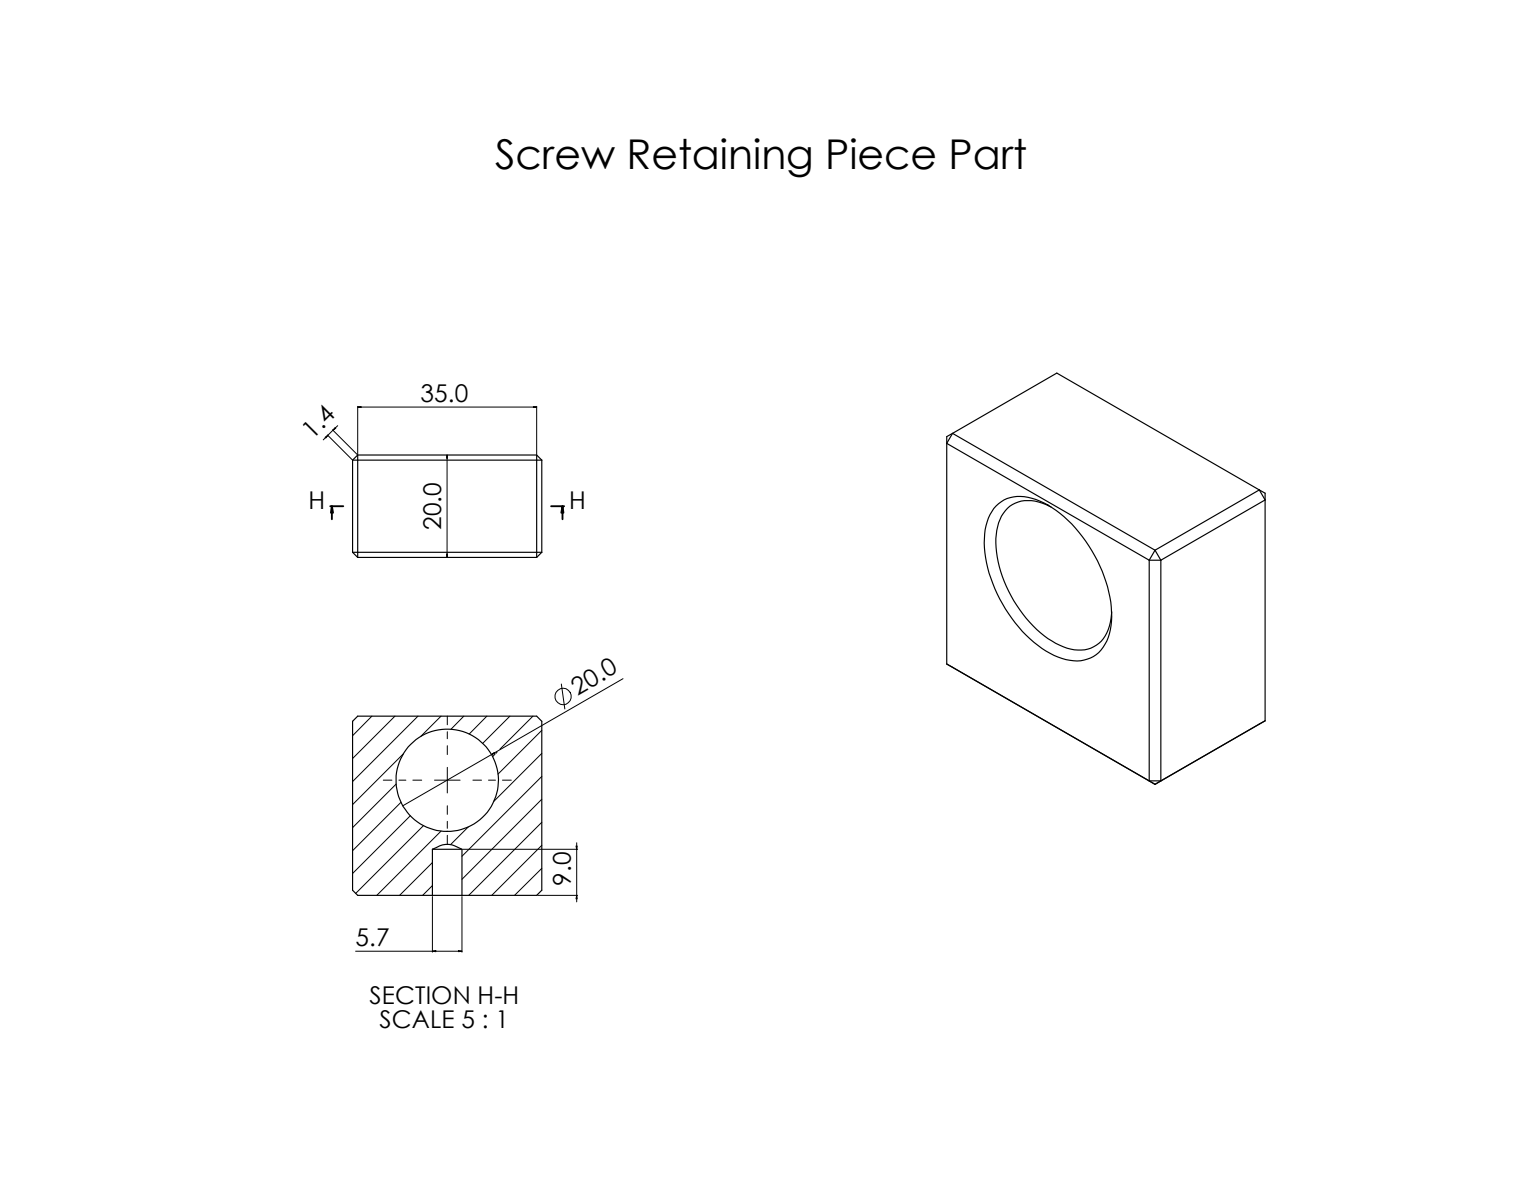
ISO-10303-21;
HEADER;
FILE_DESCRIPTION (('STEP AP214'),
    '1' );
FILE_NAME ('Screw Retaining Piece Part.step',
    '2026-10-24T22:31:37',
    ( '' ),
    ( '' ),
    'SwSTEP 2.0',
    'SolidWorks 2025',
    '' );
FILE_SCHEMA (( 'AUTOMOTIVE_DESIGN' ));
ENDSEC;

DATA;
#4=( GEOMETRIC_REPRESENTATION_CONTEXT ( 3 ) GLOBAL_UNCERTAINTY_ASSIGNED_CONTEXT ( ( #48363 ) ) GLOBAL_UNIT_ASSIGNED_CONTEXT ( ( #53726, #45627, #22843 ) ) REPRESENTATION_CONTEXT ( 'NONE', 'WORKASPACE' ) );
#17=CARTESIAN_POINT ( 'NONE',  ( 41.47569090598248920, 209.1868197944957899, -17.47570218321533631 ) ) ;
#445=VECTOR ( 'NONE', #6291, 1000.000000000000000 ) ;
#696=ORIENTED_EDGE ( 'NONE', *, *, #30280, .F. ) ;
#887=DIRECTION ( 'NONE',  ( 0.6123724356958057946, 0.3535533905932591314, 0.7071067811865451302 ) ) ;
#1022=DIRECTION ( 'NONE',  ( 0.2588190451025028094, 0.9659258262890731972, -2.513112717808992705E-15 ) ) ;
#1048=CARTESIAN_POINT ( 'NONE',  ( 80.00798602660123038, 150.6044130683315814, 4.041334437186263538E-16 ) ) ;
#1205=FACE_OUTER_BOUND ( 'NONE', #66271, .T. ) ;
#1327=PLANE ( 'NONE',  #96927 ) ;
#1361=VERTEX_POINT ( 'NONE', #15363 ) ;
#1362=DIRECTION ( 'NONE',  ( -0.2588190451025239591, -0.9659258262890673130, -6.568581106066860352E-16 ) ) ;
#1612=VECTOR ( 'NONE', #92271, 1000.000000000000114 ) ;
#1651=PLANE ( 'NONE',  #2903 ) ;
#1667=EDGE_CURVE ( 'NONE', #92124, #12322, #84217, .T. ) ;
#1773=UNCERTAINTY_MEASURE_WITH_UNIT (LENGTH_MEASURE( 1.000000000000000082E-05 ), #86839, 'distance_accuracy_value', 'NONE');
#1975=CARTESIAN_POINT ( 'NONE',  ( 46.85966550219794158, 197.8615022471903728, 4.537668576076727938E-14 ) ) ;
#1997=VERTEX_POINT ( 'NONE', #7665 ) ;
#2024=CARTESIAN_POINT ( 'NONE',  ( 41.10966550219799842, 207.8207943907112281, 18.47570218321542868 ) ) ;
#2083=ORIENTED_EDGE ( 'NONE', *, *, #56810, .T. ) ;
#2086=ORIENTED_EDGE ( 'NONE', *, *, #49860, .T. ) ;
#2096=VERTEX_POINT ( 'NONE', #31283 ) ;
#2672=DIRECTION ( 'NONE',  ( 0.3535533905932688459, -0.6123724356957851445, -0.7071067811865581199 ) ) ;
#2699=EDGE_CURVE ( 'NONE', #82304, #55615, #96400, .T. ) ;
#2702=VECTOR ( 'NONE', #64696, 1000.000000000000227 ) ;
#2733=EDGE_CURVE ( 'NONE', #23710, #48945, #91778, .T. ) ;
#2851=CARTESIAN_POINT ( 'NONE',  ( 58.97569090598251051, 178.8759306620404175, -18.47570218321542868 ) ) ;
#2903=AXIS2_PLACEMENT_3D ( 'NONE', #63430, #94368, #55797 ) ;
#2965=AXIS2_PLACEMENT_3D ( 'NONE', #13155, #7022, #6539 ) ;
#3120=CIRCLE ( 'NONE', #62712, 9.999999999999998224 ) ;
#3217=EDGE_CURVE ( 'NONE', #33352, #52344, #30328, .T. ) ;
#3493=ORIENTED_EDGE ( 'NONE', *, *, #23976, .F. ) ;
#3575=VECTOR ( 'NONE', #23234, 1000.000000000000227 ) ;
#3771=CARTESIAN_POINT ( 'NONE',  ( 74.56414817410228579, 187.8759306620403322, -17.47570218321536117 ) ) ;
#3795=VECTOR ( 'NONE', #10139, 1000.000000000000227 ) ;
#3868=FACE_OUTER_BOUND ( 'NONE', #21734, .T. ) ;
#4007=EDGE_CURVE ( 'NONE', #52344, #77213, #15126, .T. ) ;
#4098=LINE ( 'NONE', #81153, #83476 ) ;
#4141=LINE ( 'NONE', #79698, #48062 ) ;
#4360=DIRECTION ( 'NONE',  ( 0.000000000000000000, 0.000000000000000000, -1.000000000000000000 ) ) ;
#4588=CARTESIAN_POINT ( 'NONE',  ( 57.60966550219794158, 179.2419560658248940, -18.47570218321542868 ) ) ;
#4714=EDGE_CURVE ( 'NONE', #59587, #2096, #71626, .T. ) ;
#4726=ORIENTED_EDGE ( 'NONE', *, *, #13893, .T. ) ;
#4763=DIRECTION ( 'NONE',  ( 0.8660254037844363761, 0.5000000000000039968, 0.000000000000000000 ) ) ;
#4843=ADVANCED_FACE ( 'NONE', ( #98367, #90798 ), #22832, .F. ) ;
#4855=DIRECTION ( 'NONE',  ( -0.5906904945688551400, 0.000000000000000000, 0.8068982213550859317 ) ) ;
#4970=DIRECTION ( 'NONE',  ( 0.000000000000000000, -0.5906904945688906672, 0.8068982213550599525 ) ) ;
#5066=EDGE_LOOP ( 'NONE', ( #50417, #33111 ) ) ;
#5094=DIRECTION ( 'NONE',  ( -0.6123724356957859216, -0.3535533905932690124, 0.7071067811865573427 ) ) ;
#5255=EDGE_CURVE ( 'NONE', #1997, #61284, #67583, .T. ) ;
#5310=CARTESIAN_POINT ( 'NONE',  ( 138.1418008908465822, 79.75620593067000641, 17.47570218321536473 ) ) ;
#5572=ORIENTED_EDGE ( 'NONE', *, *, #25630, .F. ) ;
#5684=ORIENTED_EDGE ( 'NONE', *, *, #3217, .F. ) ;
#5791=EDGE_CURVE ( 'NONE', #55615, #92124, #97769, .T. ) ;
#5804=DIRECTION ( 'NONE',  ( 0.8660254037844382635, 0.5000000000000004441, 0.000000000000000000 ) ) ;
#5829=CARTESIAN_POINT ( 'NONE',  ( 41.47569090598248920, 209.1868197944957899, -17.47570218321533631 ) ) ;
#5965=DIRECTION ( 'NONE',  ( -0.6123724356958019088, -0.3535533905932806698, -0.7071067811865376918 ) ) ;
#6187=ORIENTED_EDGE ( 'NONE', *, *, #36829, .T. ) ;
#6291=DIRECTION ( 'NONE',  ( -2.816764622163176999E-16, -1.626259812849726945E-16, 1.000000000000000000 ) ) ;
#6347=EDGE_CURVE ( 'NONE', #70099, #22001, #39787, .T. ) ;
#6351=FACE_OUTER_BOUND ( 'NONE', #68131, .T. ) ;
#6538=DIRECTION ( 'NONE',  ( -0.3535533905933014309, 0.6123724356957908066, -0.7071067811865369146 ) ) ;
#6539=DIRECTION ( 'NONE',  ( -0.8660254037844382635, -0.5000000000000004441, 0.000000000000000000 ) ) ;
#6835=CARTESIAN_POINT ( 'NONE',  ( 74.56414817410228579, 187.8759306620403322, -18.47570218321542868 ) ) ;
#6869=VECTOR ( 'NONE', #99259, 1000.000000000000227 ) ;
#6872=CARTESIAN_POINT ( 'NONE',  ( 74.06414817410220053, 188.7419560658248656, 18.47570218321542868 ) ) ;
#6898=ORIENTED_EDGE ( 'NONE', *, *, #46398, .F. ) ;
#7022=DIRECTION ( 'NONE',  ( -0.5000000000000005551, 0.8660254037844383745, -1.877843081442120711E-16 ) ) ;
#7154=VERTEX_POINT ( 'NONE', #67416 ) ;
#7343=EDGE_CURVE ( 'NONE', #19698, #52344, #15704, .T. ) ;
#7409=EDGE_CURVE ( 'NONE', #27141, #91686, #64317, .T. ) ;
#7413=DIRECTION ( 'NONE',  ( 0.3535533905932811694, -0.6123724356958052395, 0.7071067811865344721 ) ) ;
#7461=ADVANCED_FACE ( 'NONE', ( #17728, #33939 ), #72445, .T. ) ;
#7616=LINE ( 'NONE', #2024, #1612 ) ;
#7665=CARTESIAN_POINT ( 'NONE',  ( 74.56414817410228579, 187.8759306620403322, -17.47570218321536473 ) ) ;
#7687=CARTESIAN_POINT ( 'NONE',  ( 74.56414817410227158, 187.8759306620403322, 17.47570218321536473 ) ) ;
#7788=ADVANCED_FACE ( 'NONE', ( #95802 ), #81583, .F. ) ;
#7804=CARTESIAN_POINT ( 'NONE',  ( 58.43017357788679789, 217.8207943907112849, 2.194453944013935930E-14 ) ) ;
#7845=ORIENTED_EDGE ( 'NONE', *, *, #25758, .T. ) ;
#7942=EDGE_LOOP ( 'NONE', ( #41453, #80243, #46344, #86963 ) ) ;
#8056=ORIENTED_EDGE ( 'NONE', *, *, #58512, .F. ) ;
#8193=DIRECTION ( 'NONE',  ( 0.3535533905932853882, -0.6123724356958029080, -0.7071067811865343611 ) ) ;
#8195=CARTESIAN_POINT ( 'NONE',  ( 64.18017357788670552, 207.8615022471903728, 5.188172501216618598E-14 ) ) ;
#8263=PLANE ( 'NONE',  #42604 ) ;
#8421=CARTESIAN_POINT ( 'NONE',  ( 74.49716087599448144, 188.9919560658248656, 17.97570218321540381 ) ) ;
#8813=ORIENTED_EDGE ( 'NONE', *, *, #20301, .F. ) ;
#8987=CARTESIAN_POINT ( 'NONE',  ( 40.60966550219798421, 208.6868197944957615, 17.47570218321536117 ) ) ;
#9164=DIRECTION ( 'NONE',  ( 0.8660254037844384856, 0.5000000000000002220, 3.252519625699449945E-16 ) ) ;
#9259=CIRCLE ( 'NONE', #72421, 3.299999999999998934 ) ;
#9375=CIRCLE ( 'NONE', #66002, 10.99999999999999112 ) ;
#9419=CARTESIAN_POINT ( 'NONE',  ( 41.47569090598248920, 209.1868197944957899, -18.47570218321542868 ) ) ;
#9464=LINE ( 'NONE', #71776, #11066 ) ;
#9475=ORIENTED_EDGE ( 'NONE', *, *, #36829, .F. ) ;
#9550=ORIENTED_EDGE ( 'NONE', *, *, #21528, .F. ) ;
#9684=CARTESIAN_POINT ( 'NONE',  ( 41.10966550219798421, 207.8207943907112565, -18.47570218321542868 ) ) ;
#9725=CARTESIAN_POINT ( 'NONE',  ( 57.60966550219797000, 179.2419560658249225, 17.47570218321536117 ) ) ;
#9846=EDGE_CURVE ( 'NONE', #33352, #92124, #99612, .T. ) ;
#9941=ORIENTED_EDGE ( 'NONE', *, *, #6347, .T. ) ;
#10082=LINE ( 'NONE', #47070, #75361 ) ;
#10139=DIRECTION ( 'NONE',  ( 0.5000000000000002220, -0.8660254037844384856, 0.000000000000000000 ) ) ;
#10171=CARTESIAN_POINT ( 'NONE',  ( -0.1018587248682858715, 159.2012482093460051, 2.708621480571796156E-14 ) ) ;
#10195=ORIENTED_EDGE ( 'NONE', *, *, #5255, .F. ) ;
#10254=VERTEX_POINT ( 'NONE', #73694 ) ;
#10290=CLOSED_SHELL ( 'NONE', ( #99146, #17233, #42355, #7788, #32345, #25198, #64168, #20836, #38012, #4843, #7461, #23647, #47207, #58681, #48831, #29101, #62125, #99445, #19783, #31770, #44757, #76174, #44827, #71010, #95613, #31885, #77143, #65931, #22488, #66205, #73309, #54693, #94780, #22651, #64753, #51910 ) ) ;
#10354=ORIENTED_EDGE ( 'NONE', *, *, #72324, .F. ) ;
#10431=PLANE ( 'NONE',  #98626 ) ;
#10436=PLANE ( 'NONE',  #91855 ) ;
#10583=DIRECTION ( 'NONE',  ( 0.6123724356957949144, 0.3535533905933026522, -0.7071067811865326957 ) ) ;
#10671=DIRECTION ( 'NONE',  ( -0.6123724356957797044, -0.3535533905932748411, 0.7071067811865598962 ) ) ;
#10787=( NAMED_UNIT ( * ) SI_UNIT ( $, .STERADIAN. ) SOLID_ANGLE_UNIT ( ) );
#10898=MANIFOLD_SOLID_BREP ( 'Chamfer4', #10290 ) ;
#10926=ORIENTED_EDGE ( 'NONE', *, *, #77533, .F. ) ;
#11066=VECTOR ( 'NONE', #18068, 1000.000000000000000 ) ;
#11131=VECTOR ( 'NONE', #49638, 1000.000000000000114 ) ;
#11140=CARTESIAN_POINT ( 'NONE',  ( 58.31414817410232843, 216.0217562850347690, 5.155647304959626021E-14 ) ) ;
#11143=DIRECTION ( 'NONE',  ( -0.2588190451025115801, -0.9659258262890707547, -2.299878683274414842E-16 ) ) ;
#11174=LINE ( 'NONE', #19278, #11131 ) ;
#11326=LINE ( 'NONE', #41682, #36992 ) ;
#11451=DIRECTION ( 'NONE',  ( -0.6123724356958050175, -0.3535533905932800591, -0.7071067811865352493 ) ) ;
#11557=FACE_OUTER_BOUND ( 'NONE', #50919, .T. ) ;
#11741=PLANE ( 'NONE',  #20670 ) ;
#11778=DIRECTION ( 'NONE',  ( -0.9659258262890627611, 0.2588190451025410010, -1.722766911950497786E-15 ) ) ;
#12047=PLANE ( 'NONE',  #46677 ) ;
#12113=AXIS2_PLACEMENT_3D ( 'NONE', #9725, #25917, #40579 ) ;
#12152=CARTESIAN_POINT ( 'NONE',  ( 82.86586985908988368, 152.2544130683315871, 0.000000000000000000 ) ) ;
#12306=VERTEX_POINT ( 'NONE', #76300 ) ;
#12322=VERTEX_POINT ( 'NONE', #6872 ) ;
#12540=ORIENTED_EDGE ( 'NONE', *, *, #32497, .T. ) ;
#12552=DIRECTION ( 'NONE',  ( -0.5000000000000002220, 0.8660254037844384856, 0.000000000000000000 ) ) ;
#12630=LINE ( 'NONE', #49613, #83569 ) ;
#12683=EDGE_CURVE ( 'NONE', #12306, #80748, #94264, .T. ) ;
#12749=VECTOR ( 'NONE', #67040, 1000.000000000000114 ) ;
#12815=ORIENTED_EDGE ( 'NONE', *, *, #12683, .T. ) ;
#12877=DIRECTION ( 'NONE',  ( -0.5000000000000019984, 0.8660254037844374864, 0.000000000000000000 ) ) ;
#12983=EDGE_LOOP ( 'NONE', ( #25152, #72504, #13340, #57946 ) ) ;
#13155=CARTESIAN_POINT ( 'NONE',  ( 40.60966550219796289, 208.6868197944957330, -18.47570218321542868 ) ) ;
#13227=EDGE_CURVE ( 'NONE', #1997, #97187, #33673, .T. ) ;
#13245=EDGE_CURVE ( 'NONE', #15824, #22001, #19968, .T. ) ;
#13340=ORIENTED_EDGE ( 'NONE', *, *, #36398, .T. ) ;
#13419=DIRECTION ( 'NONE',  ( -0.6123724356957817028, -0.3535533905932665699, -0.7071067811865623387 ) ) ;
#13471=LINE ( 'NONE', #91994, #33247 ) ;
#13559=ORIENTED_EDGE ( 'NONE', *, *, #96924, .F. ) ;
#13637=PRODUCT ( 'Screw Retaining Piece Part', 'Screw Retaining Piece Part', '', ( #36050 ) ) ;
#13893=EDGE_CURVE ( 'NONE', #15824, #7154, #48643, .T. ) ;
#14246=DIRECTION ( 'NONE',  ( -0.5000000000000002220, 0.8660254037844384856, 0.000000000000000000 ) ) ;
#14270=CARTESIAN_POINT ( 'NONE',  ( 57.60966550219794158, 179.2419560658248940, 18.47570218321542868 ) ) ;
#14403=CARTESIAN_POINT ( 'NONE',  ( 58.43017357788678368, 217.8207943907113133, 2.194453944013934668E-14 ) ) ;
#14708=ORIENTED_EDGE ( 'NONE', *, *, #13245, .T. ) ;
#14923=LINE ( 'NONE', #6835, #91039 ) ;
#14940=VERTEX_POINT ( 'NONE', #72732 ) ;
#15126=LINE ( 'NONE', #75983, #3575 ) ;
#15194=DIRECTION ( 'NONE',  ( 0.3535533905932665699, -0.6123724356957869208, -0.7071067811865576758 ) ) ;
#15354=CARTESIAN_POINT ( 'NONE',  ( 0.000000000000000000, 0.000000000000000000, 0.000000000000000000 ) ) ;
#15363=CARTESIAN_POINT ( 'NONE',  ( 57.56414817410227869, 217.3207943907111996, 18.47570218321542868 ) ) ;
#15540=EDGE_LOOP ( 'NONE', ( #21084, #10354, #27539, #8056 ) ) ;
#15704=LINE ( 'NONE', #77536, #33573 ) ;
#15752=DIRECTION ( 'NONE',  ( 0.8660254037844385966, 0.5000000000000002220, 3.252519625699450438E-16 ) ) ;
#15776=LINE ( 'NONE', #7687, #27252 ) ;
#15824=VERTEX_POINT ( 'NONE', #20489 ) ;
#16071=ORIENTED_EDGE ( 'NONE', *, *, #7409, .T. ) ;
#16310=EDGE_LOOP ( 'NONE', ( #56375, #26252, #12815, #94819 ) ) ;
#17233=ADVANCED_FACE ( 'NONE', ( #27573 ), #59339, .F. ) ;
#17273=CARTESIAN_POINT ( 'NONE',  ( 68.22375369157857961, 184.2153022007868515, 0.000000000000000000 ) ) ;
#17428=ORIENTED_EDGE ( 'NONE', *, *, #4714, .F. ) ;
#17525=DIRECTION ( 'NONE',  ( -0.3535533905932676246, 0.6123724356957830350, -0.7071067811865604513 ) ) ;
#17601=DIRECTION ( 'NONE',  ( 0.5000000000000002220, -0.8660254037844387076, -0.000000000000000000 ) ) ;
#17602=DIRECTION ( 'NONE',  ( -0.6123724356958113457, -0.3535533905932644605, -0.7071067811865376918 ) ) ;
#17728=FACE_BOUND ( 'NONE', #39307, .T. ) ;
#17857=EDGE_CURVE ( 'NONE', #59587, #27141, #43493, .T. ) ;
#17925=ORIENTED_EDGE ( 'NONE', *, *, #65535, .T. ) ;
#18035=ORIENTED_EDGE ( 'NONE', *, *, #46398, .T. ) ;
#18068=DIRECTION ( 'NONE',  ( -2.816764622163176506E-16, -1.626259812849726205E-16, 1.000000000000000000 ) ) ;
#18595=LINE ( 'NONE', #26188, #72685 ) ;
#18756=ORIENTED_EDGE ( 'NONE', *, *, #21223, .T. ) ;
#18757=DIRECTION ( 'NONE',  ( 0.5000000000000001110, -0.8660254037844384856, -0.000000000000000000 ) ) ;
#18805=DIRECTION ( 'NONE',  ( -0.5000000000000002220, 0.8660254037844384856, 0.000000000000000000 ) ) ;
#18809=EDGE_LOOP ( 'NONE', ( #10926, #45886, #28773, #6898 ) ) ;
#18878=CONICAL_SURFACE ( 'NONE', #99792, 3.299999999999978950, 1.029744258676652313 ) ;
#19228=EDGE_CURVE ( 'NONE', #1361, #33352, #7616, .T. ) ;
#19278=CARTESIAN_POINT ( 'NONE',  ( 41.10966550219798421, 207.8207943907112565, -18.47570218321542868 ) ) ;
#19488=CARTESIAN_POINT ( 'NONE',  ( 65.36586985908992631, 182.5653022007868458, 0.000000000000000000 ) ) ;
#19671=EDGE_CURVE ( 'NONE', #12306, #14940, #78632, .T. ) ;
#19686=ORIENTED_EDGE ( 'NONE', *, *, #4007, .T. ) ;
#19698=VERTEX_POINT ( 'NONE', #80448 ) ;
#19783=ADVANCED_FACE ( 'NONE', ( #60068 ), #99104, .T. ) ;
#19791=LINE ( 'NONE', #81611, #59615 ) ;
#19941=ORIENTED_EDGE ( 'NONE', *, *, #36136, .F. ) ;
#19949=ORIENTED_EDGE ( 'NONE', *, *, #37503, .F. ) ;
#19968=LINE ( 'NONE', #20468, #48379 ) ;
#20076=CARTESIAN_POINT ( 'NONE',  ( 58.10966550219799132, 178.3759306620403606, -18.47570218321542868 ) ) ;
#20095=DIRECTION ( 'NONE',  ( 0.3535533905932783383, -0.6123724356958041293, 0.7071067811865369146 ) ) ;
#20173=CARTESIAN_POINT ( 'NONE',  ( 58.43017357788679789, 217.8207943907112849, 17.47570218321536117 ) ) ;
#20301=EDGE_CURVE ( 'NONE', #74475, #12306, #26963, .T. ) ;
#20468=CARTESIAN_POINT ( 'NONE',  ( 41.47569090598248920, 209.1868197944957899, -17.47570218321533631 ) ) ;
#20489=CARTESIAN_POINT ( 'NONE',  ( 41.10966550219804816, 207.8207943907112565, -17.47570218321534696 ) ) ;
#20531=EDGE_CURVE ( 'NONE', #1361, #45554, #10082, .T. ) ;
#20559=AXIS2_PLACEMENT_3D ( 'NONE', #26068, #58440, #12877 ) ;
#20670=AXIS2_PLACEMENT_3D ( 'NONE', #26441, #51206, #89290 ) ;
#20684=VERTEX_POINT ( 'NONE', #43832 ) ;
#20711=DIRECTION ( 'NONE',  ( 2.816764622163176506E-16, 1.626259812849726698E-16, -1.000000000000000000 ) ) ;
#20821=ORIENTED_EDGE ( 'NONE', *, *, #25371, .T. ) ;
#20836=ADVANCED_FACE ( 'NONE', ( #20944 ), #42702, .T. ) ;
#20944=FACE_OUTER_BOUND ( 'NONE', #52756, .T. ) ;
#20949=CARTESIAN_POINT ( 'NONE',  ( 60.86586985908987657, 190.3595308348468791, 0.000000000000000000 ) ) ;
#21059=FACE_OUTER_BOUND ( 'NONE', #72272, .T. ) ;
#21084=ORIENTED_EDGE ( 'NONE', *, *, #13227, .F. ) ;
#21223=EDGE_CURVE ( 'NONE', #76155, #81724, #4098, .T. ) ;
#21407=DIRECTION ( 'NONE',  ( 0.2113248654051647635, 0.7886751345948180836, -0.5773502691896270633 ) ) ;
#21528=EDGE_CURVE ( 'NONE', #82304, #92124, #63165, .T. ) ;
#21642=PRODUCT_DEFINITION ( 'UNKNOWN', '', #83512, #78771 ) ;
#21734=EDGE_LOOP ( 'NONE', ( #46283, #73198, #57401, #51411 ) ) ;
#21843=CIRCLE ( 'NONE', #67185, 10.99999999999999112 ) ;
#21868=FACE_OUTER_BOUND ( 'NONE', #12983, .T. ) ;
#21878=ORIENTED_EDGE ( 'NONE', *, *, #4007, .F. ) ;
#22001=VERTEX_POINT ( 'NONE', #17 ) ;
#22057=ORIENTED_EDGE ( 'NONE', *, *, #71081, .F. ) ;
#22488=ADVANCED_FACE ( 'NONE', ( #28247 ), #98678, .T. ) ;
#22541=DIRECTION ( 'NONE',  ( 0.5000000000000002220, -0.8660254037844385966, 0.000000000000000000 ) ) ;
#22651=ADVANCED_FACE ( 'NONE', ( #21059 ), #66137, .T. ) ;
#22666=CARTESIAN_POINT ( 'NONE',  ( 57.56414817410229290, 217.3207943907112281, -18.47570218321543223 ) ) ;
#22832=PLANE ( 'NONE',  #31153 ) ;
#22837=CARTESIAN_POINT ( 'NONE',  ( 68.31414817410235685, 198.7012482093460335, 5.278111984874361800E-14 ) ) ;
#22843=( NAMED_UNIT ( * ) SI_UNIT ( $, .STERADIAN. ) SOLID_ANGLE_UNIT ( ) );
#23119=ORIENTED_EDGE ( 'NONE', *, *, #37709, .T. ) ;
#23136=VECTOR ( 'NONE', #6538, 1000.000000000000000 ) ;
#23234=DIRECTION ( 'NONE',  ( 0.8660254037844382635, 0.5000000000000004441, 1.232595164407830946E-32 ) ) ;
#23377=CARTESIAN_POINT ( 'NONE',  ( 74.93017357788676236, 189.2419560658248940, -17.47570218321535052 ) ) ;
#23457=DIRECTION ( 'NONE',  ( 1.000000000000000000, 0.000000000000000000, 0.000000000000000000 ) ) ;
#23534=ORIENTED_EDGE ( 'NONE', *, *, #70529, .F. ) ;
#23647=ADVANCED_FACE ( 'NONE', ( #6351 ), #18878, .F. ) ;
#23710=VERTEX_POINT ( 'NONE', #70118 ) ;
#23756=ORIENTED_EDGE ( 'NONE', *, *, #49860, .F. ) ;
#23795=CARTESIAN_POINT ( 'NONE',  ( 58.97569090598253183, 178.8759306620404175, -18.47570218321542868 ) ) ;
#23914=VECTOR ( 'NONE', #49644, 1000.000000000000000 ) ;
#23976=EDGE_CURVE ( 'NONE', #77213, #45554, #96704, .T. ) ;
#24152=ORIENTED_EDGE ( 'NONE', *, *, #5791, .F. ) ;
#24366=LINE ( 'NONE', #72493, #98645 ) ;
#24625=ORIENTED_EDGE ( 'NONE', *, *, #20531, .T. ) ;
#24644=CARTESIAN_POINT ( 'NONE',  ( 74.56414817410228579, 187.8759306620403322, -17.47570218321536473 ) ) ;
#24682=CARTESIAN_POINT ( 'NONE',  ( 41.54267820409027223, 208.0707943907112565, 17.97570218321537538 ) ) ;
#24756=VECTOR ( 'NONE', #47897, 1000.000000000000114 ) ;
#25037=CONICAL_SURFACE ( 'NONE', #86567, 11.00000000000002842, 0.7853981633974557175 ) ;
#25149=VECTOR ( 'NONE', #64171, 1000.000000000000000 ) ;
#25152=ORIENTED_EDGE ( 'NONE', *, *, #4714, .T. ) ;
#25193=LINE ( 'NONE', #87070, #54430 ) ;
#25198=ADVANCED_FACE ( 'NONE', ( #3868 ), #65653, .T. ) ;
#25311=CARTESIAN_POINT ( 'NONE',  ( 138.1418008908465822, 79.75620593067000641, 5.188172501216618598E-14 ) ) ;
#25371=EDGE_CURVE ( 'NONE', #19698, #15824, #13471, .T. ) ;
#25476=SHAPE_REPRESENTATION_RELATIONSHIP ( 'NONE' , 'NONE' ,  #94304, #88828 ) ;
#25630=EDGE_CURVE ( 'NONE', #74475, #14940, #41730, .T. ) ;
#25729=DIRECTION ( 'NONE',  ( -0.8660254037844379305, -0.5000000000000016653, -3.252519625699479034E-16 ) ) ;
#25758=EDGE_CURVE ( 'NONE', #22001, #52344, #70516, .T. ) ;
#25872=FACE_OUTER_BOUND ( 'NONE', #39798, .T. ) ;
#25917=DIRECTION ( 'NONE',  ( -0.2113248654052032327, -0.7886751345948027625, 0.5773502691896338357 ) ) ;
#26068=CARTESIAN_POINT ( 'NONE',  ( 63.31414817410234264, 207.3615022471904012, 5.155647304959626021E-14 ) ) ;
#26188=CARTESIAN_POINT ( 'NONE',  ( 57.31414817410225027, 217.7538070926034379, 17.97570218321539315 ) ) ;
#26244=PLANE ( 'NONE',  #95345 ) ;
#26252=ORIENTED_EDGE ( 'NONE', *, *, #19671, .F. ) ;
#26365=LINE ( 'NONE', #57240, #23914 ) ;
#26441=CARTESIAN_POINT ( 'NONE',  ( 41.47569090598247499, 209.1868197944957899, 17.47570218321535762 ) ) ;
#26554=CARTESIAN_POINT ( 'NONE',  ( 58.00798602660123748, 188.7095308348469018, 4.041334437186252691E-16 ) ) ;
#26569=DIRECTION ( 'NONE',  ( 0.2588190451025027539, 0.9659258262890731972, 6.846136862223680982E-16 ) ) ;
#26675=VECTOR ( 'NONE', #33205, 999.9999999999998863 ) ;
#26799=DIRECTION ( 'NONE',  ( -0.8660254037844384856, -0.5000000000000002220, -3.252519625699449945E-16 ) ) ;
#26963=LINE ( 'NONE', #99233, #96780 ) ;
#27063=DIRECTION ( 'NONE',  ( 0.5000000000000005551, -0.8660254037844384856, 0.000000000000000000 ) ) ;
#27121=AXIS2_PLACEMENT_3D ( 'NONE', #91630, #30297, #84048 ) ;
#27141=VERTEX_POINT ( 'NONE', #58656 ) ;
#27191=AXIS2_PLACEMENT_3D ( 'NONE', #67808, #59174, #51609 ) ;
#27252=VECTOR ( 'NONE', #8193, 1000.000000000000114 ) ;
#27253=AXIS2_PLACEMENT_3D ( 'NONE', #29015, #21407, #37576 ) ;
#27273=CARTESIAN_POINT ( 'NONE',  ( 58.43017357788679789, 217.8207943907112849, 17.47570218321536473 ) ) ;
#27303=DIRECTION ( 'NONE',  ( -0.4999999999999996669, 0.8660254037844387076, 0.000000000000000000 ) ) ;
#27539=ORIENTED_EDGE ( 'NONE', *, *, #96408, .F. ) ;
#27573=FACE_OUTER_BOUND ( 'NONE', #47614, .T. ) ;
#27676=EDGE_LOOP ( 'NONE', ( #52775, #18035 ) ) ;
#27746=DIRECTION ( 'NONE',  ( 0.8660254037844384856, 0.5000000000000002220, 3.252519625699449945E-16 ) ) ;
#27882=LINE ( 'NONE', #4588, #96732 ) ;
#28018=CARTESIAN_POINT ( 'NONE',  ( 58.43017357788679789, 217.8207943907112849, 17.47570218321536117 ) ) ;
#28041=EDGE_LOOP ( 'NONE', ( #2086, #88018, #73753, #96006 ) ) ;
#28159=VECTOR ( 'NONE', #94938, 999.9999999999998863 ) ;
#28247=FACE_OUTER_BOUND ( 'NONE', #92389, .T. ) ;
#28390=DIRECTION ( 'NONE',  ( 0.9659258262890730862, -0.2588190451025027539, -1.337837478769339558E-14 ) ) ;
#28552=VECTOR ( 'NONE', #74436, 1000.000000000000114 ) ;
#28616=DIRECTION ( 'NONE',  ( 0.8660254037844382635, 0.5000000000000004441, 0.000000000000000000 ) ) ;
#28773=ORIENTED_EDGE ( 'NONE', *, *, #49606, .T. ) ;
#28783=AXIS2_PLACEMENT_3D ( 'NONE', #48066, #40457, #71393 ) ;
#29008=CARTESIAN_POINT ( 'NONE',  ( 82.86586985908988368, 152.2544130683315871, 0.000000000000000000 ) ) ;
#29015=CARTESIAN_POINT ( 'NONE',  ( 57.56414817410228579, 217.3207943907112281, -18.47570218321542868 ) ) ;
#29029=DIRECTION ( 'NONE',  ( 0.000000000000000000, -0.000000000000000000, 1.000000000000000000 ) ) ;
#29101=ADVANCED_FACE ( 'NONE', ( #78485 ), #82024, .F. ) ;
#29341=PLANE ( 'NONE',  #2965 ) ;
#29344=ORIENTED_EDGE ( 'NONE', *, *, #66648, .F. ) ;
#29481=ORIENTED_EDGE ( 'NONE', *, *, #73145, .T. ) ;
#29554=ORIENTED_EDGE ( 'NONE', *, *, #34195, .F. ) ;
#29592=VECTOR ( 'NONE', #83712, 1000.000000000000114 ) ;
#29623=LINE ( 'NONE', #84357, #62800 ) ;
#29624=ORIENTED_EDGE ( 'NONE', *, *, #73145, .F. ) ;
#29819=DIRECTION ( 'NONE',  ( 0.9998476951563911586, -0.01745240643728540250, 0.000000000000000000 ) ) ;
#29967=CARTESIAN_POINT ( 'NONE',  ( -5.101858724868291617, 167.8615022471904012, 2.586156800657061008E-14 ) ) ;
#29983=DIRECTION ( 'NONE',  ( 0.8660254037844373753, 0.5000000000000021094, 0.000000000000000000 ) ) ;
#30235=VECTOR ( 'NONE', #9164, 1000.000000000000114 ) ;
#30280=EDGE_CURVE ( 'NONE', #27141, #23710, #47974, .T. ) ;
#30281=DIRECTION ( 'NONE',  ( 0.8660254037844375974, 0.5000000000000017764, 3.252519625699413953E-16 ) ) ;
#30297=DIRECTION ( 'NONE',  ( -0.3535533905932676246, 0.6123724356957830350, 0.7071067811865604513 ) ) ;
#30328=LINE ( 'NONE', #60701, #23136 ) ;
#30329=FACE_OUTER_BOUND ( 'NONE', #32865, .T. ) ;
#30630=VECTOR ( 'NONE', #43119, 1000.000000000000227 ) ;
#30796=LINE ( 'NONE', #24682, #57283 ) ;
#31007=DIRECTION ( 'NONE',  ( 0.8660254037844363761, 0.5000000000000039968, 0.000000000000000000 ) ) ;
#31085=DIRECTION ( 'NONE',  ( -0.2588190451025027539, -0.9659258262890730862, -9.720431063823805450E-17 ) ) ;
#31089=CARTESIAN_POINT ( 'NONE',  ( 74.93017357788674815, 189.2419560658248940, 17.47570218321536117 ) ) ;
#31150=DIRECTION ( 'NONE',  ( -0.5000000000000019984, 0.8660254037844374864, 0.000000000000000000 ) ) ;
#31153=AXIS2_PLACEMENT_3D ( 'NONE', #84677, #83685, #14246 ) ;
#31283=CARTESIAN_POINT ( 'NONE',  ( 52.72569090598241104, 189.7012482093459766, 4.692658452248458818E-14 ) ) ;
#31459=ORIENTED_EDGE ( 'NONE', *, *, #7409, .F. ) ;
#31485=EDGE_LOOP ( 'NONE', ( #88479, #99763, #87898, #58493 ) ) ;
#31550=LINE ( 'NONE', #48266, #64402 ) ;
#31770=ADVANCED_FACE ( 'NONE', ( #77650 ), #1651, .T. ) ;
#31883=ORIENTED_EDGE ( 'NONE', *, *, #19228, .F. ) ;
#31885=ADVANCED_FACE ( 'NONE', ( #97841 ), #11741, .T. ) ;
#31892=EDGE_LOOP ( 'NONE', ( #98515, #96360, #86637, #58760 ) ) ;
#32159=DIRECTION ( 'NONE',  ( 0.8660254037844375974, 0.5000000000000017764, 3.252519625699413953E-16 ) ) ;
#32208=DIRECTION ( 'NONE',  ( -0.9659258262890730862, 0.2588190451025027539, -3.627714260166394782E-16 ) ) ;
#32222=ORIENTED_EDGE ( 'NONE', *, *, #81676, .T. ) ;
#32345=ADVANCED_FACE ( 'NONE', ( #84534 ), #41689, .F. ) ;
#32347=ORIENTED_EDGE ( 'NONE', *, *, #76478, .F. ) ;
#32497=EDGE_CURVE ( 'NONE', #78822, #1997, #71773, .T. ) ;
#32724=EDGE_LOOP ( 'NONE', ( #90819, #50080, #74090, #6187 ) ) ;
#32865=EDGE_LOOP ( 'NONE', ( #51881, #91068, #7845, #19686 ) ) ;
#32952=DIRECTION ( 'NONE',  ( 0.8660254037844382635, 0.5000000000000004441, 0.000000000000000000 ) ) ;
#32955=ORIENTED_EDGE ( 'NONE', *, *, #77533, .T. ) ;
#33040=CARTESIAN_POINT ( 'NONE',  ( 41.97569090598251762, 208.3207943907113133, -18.47570218321542868 ) ) ;
#33111=ORIENTED_EDGE ( 'NONE', *, *, #56810, .F. ) ;
#33205=DIRECTION ( 'NONE',  ( -0.5000000000000002220, 0.8660254037844385966, 0.000000000000000000 ) ) ;
#33247=VECTOR ( 'NONE', #45336, 1000.000000000000000 ) ;
#33352=VERTEX_POINT ( 'NONE', #60912 ) ;
#33505=FACE_OUTER_BOUND ( 'NONE', #39720, .T. ) ;
#33573=VECTOR ( 'NONE', #1022, 1000.000000000000000 ) ;
#33668=EDGE_LOOP ( 'NONE', ( #79383, #42915, #69754, #36566 ) ) ;
#33673=LINE ( 'NONE', #3771, #12749 ) ;
#33939=FACE_OUTER_BOUND ( 'NONE', #41124, .T. ) ;
#33985=CARTESIAN_POINT ( 'NONE',  ( 58.43017357788681210, 217.8207943907112849, -17.47570218321535052 ) ) ;
#34018=ORIENTED_EDGE ( 'NONE', *, *, #34195, .T. ) ;
#34129=ORIENTED_EDGE ( 'NONE', *, *, #55204, .T. ) ;
#34195=EDGE_CURVE ( 'NONE', #12322, #61284, #15776, .T. ) ;
#34350=ORIENTED_EDGE ( 'NONE', *, *, #55204, .F. ) ;
#34451=CARTESIAN_POINT ( 'NONE',  ( 46.85966550219794158, 197.8615022471903728, 4.537668576076727938E-14 ) ) ;
#34511=VECTOR ( 'NONE', #91279, 1000.000000000000227 ) ;
#34558=CARTESIAN_POINT ( 'NONE',  ( 57.60966550219797000, 179.2419560658249225, 17.47570218321535407 ) ) ;
#34654=AXIS2_PLACEMENT_3D ( 'NONE', #59163, #90137, #20711 ) ;
#34704=FACE_OUTER_BOUND ( 'NONE', #32724, .T. ) ;
#34784=CARTESIAN_POINT ( 'NONE',  ( 60.86586985908987657, 190.3595308348468791, 0.000000000000000000 ) ) ;
#34917=AXIS2_PLACEMENT_3D ( 'NONE', #34784, #17601, #96641 ) ;
#35129=DIRECTION ( 'NONE',  ( -0.4848096202463351156, -0.8746197071393968514, 1.049727191138617217E-16 ) ) ;
#35311=VERTEX_POINT ( 'NONE', #86152 ) ;
#35419=VECTOR ( 'NONE', #86683, 1000.000000000000227 ) ;
#35477=ORIENTED_EDGE ( 'NONE', *, *, #2699, .F. ) ;
#35853=DIRECTION ( 'NONE',  ( 0.2113248654051652076, 0.7886751345948035397, 0.5773502691896466033 ) ) ;
#36050=PRODUCT_CONTEXT ( 'NONE', #65412, 'mechanical' ) ;
#36136=EDGE_CURVE ( 'NONE', #91686, #48945, #80811, .T. ) ;
#36398=EDGE_CURVE ( 'NONE', #23710, #27141, #3120, .T. ) ;
#36522=EDGE_CURVE ( 'NONE', #77213, #1361, #18595, .T. ) ;
#36566=ORIENTED_EDGE ( 'NONE', *, *, #25371, .F. ) ;
#36633=VECTOR ( 'NONE', #58156, 1000.000000000000000 ) ;
#36653=CARTESIAN_POINT ( 'NONE',  ( 41.35966550219792026, 207.3877816888192172, 4.672379723982937232E-14 ) ) ;
#36734=CARTESIAN_POINT ( 'NONE',  ( 58.47569090598248209, 179.7419560658249509, 18.47570218321542868 ) ) ;
#36781=DIRECTION ( 'NONE',  ( 0.5906904945688935538, 0.000000000000000000, -0.8068982213550578431 ) ) ;
#36829=EDGE_CURVE ( 'NONE', #61284, #82304, #65203, .T. ) ;
#36992=VECTOR ( 'NONE', #72626, 1000.000000000000227 ) ;
#37085=FACE_OUTER_BOUND ( 'NONE', #16310, .T. ) ;
#37238=DIRECTION ( 'NONE',  ( 0.5000000000000001110, -0.8660254037844384856, -0.000000000000000000 ) ) ;
#37503=EDGE_CURVE ( 'NONE', #51698, #61284, #31550, .T. ) ;
#37576=DIRECTION ( 'NONE',  ( 0.000000000000000000, 0.5906904945688705721, 0.8068982213550747185 ) ) ;
#37709=EDGE_CURVE ( 'NONE', #14940, #53896, #55220, .T. ) ;
#37870=FACE_OUTER_BOUND ( 'NONE', #40047, .T. ) ;
#38012=ADVANCED_FACE ( 'NONE', ( #30329 ), #29341, .T. ) ;
#38165=DIRECTION ( 'NONE',  ( -3.755686162884236985E-16, 8.056116744242159655E-32, 1.000000000000000000 ) ) ;
#38967=ORIENTED_EDGE ( 'NONE', *, *, #9846, .F. ) ;
#39042=DIRECTION ( 'NONE',  ( -0.4999999999999997224, 0.8660254037844387076, 0.000000000000000000 ) ) ;
#39307=EDGE_LOOP ( 'NONE', ( #40645, #46901 ) ) ;
#39452=ORIENTED_EDGE ( 'NONE', *, *, #54062, .F. ) ;
#39717=VECTOR ( 'NONE', #35129, 1000.000000000000114 ) ;
#39720=EDGE_LOOP ( 'NONE', ( #35477, #62857, #24152 ) ) ;
#39787=LINE ( 'NONE', #71745, #96814 ) ;
#39798=EDGE_LOOP ( 'NONE', ( #17428, #32955, #98816, #53152 ) ) ;
#40047=EDGE_LOOP ( 'NONE', ( #73119, #10195, #60156, #97295 ) ) ;
#40457=DIRECTION ( 'NONE',  ( 0.8660254037844385966, 0.5000000000000002220, 3.252519625699450438E-16 ) ) ;
#40489=FACE_OUTER_BOUND ( 'NONE', #7942, .T. ) ;
#40579=DIRECTION ( 'NONE',  ( 0.000000000000000000, -0.5906904945688825626, -0.8068982213550659477 ) ) ;
#40645=ORIENTED_EDGE ( 'NONE', *, *, #36136, .T. ) ;
#40989=DIRECTION ( 'NONE',  ( 0.8660254037844385966, 0.5000000000000003331, 3.252519625699449945E-16 ) ) ;
#41124=EDGE_LOOP ( 'NONE', ( #76242, #69531, #98551, #47373 ) ) ;
#41453=ORIENTED_EDGE ( 'NONE', *, *, #2699, .T. ) ;
#41543=AXIS2_PLACEMENT_3D ( 'NONE', #1975, #48058, #70361 ) ;
#41554=CARTESIAN_POINT ( 'NONE',  ( 74.56414817410227158, 187.8759306620403322, 17.47570218321536473 ) ) ;
#41682=CARTESIAN_POINT ( 'NONE',  ( 40.60966550219796289, 208.6868197944957330, -17.47570218321533631 ) ) ;
#41689=CONICAL_SURFACE ( 'NONE', #49798, 3.299999999999978950, 1.029744258676652313 ) ;
#41730=LINE ( 'NONE', #26554, #39717 ) ;
#41746=EDGE_CURVE ( 'NONE', #12322, #1361, #64614, .T. ) ;
#42253=CARTESIAN_POINT ( 'NONE',  ( 58.97569090598251762, 178.8759306620404175, 17.47570218321536473 ) ) ;
#42306=DIRECTION ( 'NONE',  ( 0.5000000000000002220, -0.8660254037844384856, 0.000000000000000000 ) ) ;
#42355=ADVANCED_FACE ( 'NONE', ( #21868 ), #98893, .F. ) ;
#42415=CARTESIAN_POINT ( 'NONE',  ( 74.56414817410228579, 187.8759306620403322, -17.47570218321536473 ) ) ;
#42604=AXIS2_PLACEMENT_3D ( 'NONE', #63455, #2672, #70041 ) ;
#42630=LINE ( 'NONE', #56841, #30630 ) ;
#42702=PLANE ( 'NONE',  #94751 ) ;
#42786=FACE_BOUND ( 'NONE', #5066, .T. ) ;
#42834=DIRECTION ( 'NONE',  ( -1.000000000000000000, 0.000000000000000000, -0.000000000000000000 ) ) ;
#42915=ORIENTED_EDGE ( 'NONE', *, *, #25758, .F. ) ;
#43119=DIRECTION ( 'NONE',  ( 0.8660254037844382635, 0.5000000000000004441, 0.000000000000000000 ) ) ;
#43305=AXIS2_PLACEMENT_3D ( 'NONE', #8195, #92335, #98915 ) ;
#43421=ORIENTED_EDGE ( 'NONE', *, *, #19228, .T. ) ;
#43477=CARTESIAN_POINT ( 'NONE',  ( 64.18017357788670552, 207.8615022471903728, 5.188172501216618598E-14 ) ) ;
#43487=VECTOR ( 'NONE', #15194, 1000.000000000000000 ) ;
#43493=LINE ( 'NONE', #51606, #28552 ) ;
#43832=CARTESIAN_POINT ( 'NONE',  ( 41.35966550219792737, 207.3877816888192172, 4.672379723982937232E-14 ) ) ;
#44162=ORIENTED_EDGE ( 'NONE', *, *, #94508, .F. ) ;
#44757=ADVANCED_FACE ( 'NONE', ( #40489 ), #62282, .T. ) ;
#44827=ADVANCED_FACE ( 'NONE', ( #37870 ), #76412, .F. ) ;
#44935=EDGE_CURVE ( 'NONE', #19698, #33352, #30796, .T. ) ;
#44944=ORIENTED_EDGE ( 'NONE', *, *, #2733, .F. ) ;
#45094=EDGE_LOOP ( 'NONE', ( #18756, #53749, #80279 ) ) ;
#45331=CARTESIAN_POINT ( 'NONE',  ( 60.86586985908987657, 190.3595308348468791, 0.000000000000000000 ) ) ;
#45336=DIRECTION ( 'NONE',  ( 3.755686162884237478E-16, -5.590926415426495573E-32, -1.000000000000000000 ) ) ;
#45554=VERTEX_POINT ( 'NONE', #28018 ) ;
#45627=( NAMED_UNIT ( * ) PLANE_ANGLE_UNIT ( ) SI_UNIT ( $, .RADIAN. ) );
#45672=FACE_OUTER_BOUND ( 'NONE', #45094, .T. ) ;
#45886=ORIENTED_EDGE ( 'NONE', *, *, #99917, .F. ) ;
#46198=ORIENTED_EDGE ( 'NONE', *, *, #44935, .F. ) ;
#46283=ORIENTED_EDGE ( 'NONE', *, *, #70529, .T. ) ;
#46344=ORIENTED_EDGE ( 'NONE', *, *, #60318, .F. ) ;
#46396=ORIENTED_EDGE ( 'NONE', *, *, #96408, .T. ) ;
#46398=EDGE_CURVE ( 'NONE', #20684, #89824, #21843, .T. ) ;
#46402=LINE ( 'NONE', #83971, #49218 ) ;
#46554=EDGE_LOOP ( 'NONE', ( #73114, #38967, #46198, #39452 ) ) ;
#46677=AXIS2_PLACEMENT_3D ( 'NONE', #42415, #73349, #66238 ) ;
#46709=DIRECTION ( 'NONE',  ( 0.5000000000000005551, -0.8660254037844384856, 0.000000000000000000 ) ) ;
#46858=DIRECTION ( 'NONE',  ( 0.8660254037844375974, 0.5000000000000017764, 3.252519625699413953E-16 ) ) ;
#46901=ORIENTED_EDGE ( 'NONE', *, *, #58424, .T. ) ;
#47070=CARTESIAN_POINT ( 'NONE',  ( 58.43017357788679789, 217.8207943907112849, 17.47570218321536473 ) ) ;
#47100=ORIENTED_EDGE ( 'NONE', *, *, #23976, .T. ) ;
#47207=ADVANCED_FACE ( 'NONE', ( #37085 ), #68976, .F. ) ;
#47373=ORIENTED_EDGE ( 'NONE', *, *, #71081, .T. ) ;
#47614=EDGE_LOOP ( 'NONE', ( #55692, #70882, #19941, #31459 ) ) ;
#47684=CARTESIAN_POINT ( 'NONE',  ( 59.87444983769439943, 192.0767206835448633, -1.126254757482173519E-14 ) ) ;
#47897=DIRECTION ( 'NONE',  ( 0.6123724356958143433, 0.3535533905932691234, -0.7071067811865326957 ) ) ;
#47905=VECTOR ( 'NONE', #5965, 1000.000000000000000 ) ;
#47951=CARTESIAN_POINT ( 'NONE',  ( 58.72569090598248920, 179.3089433639326842, 17.97570218321541446 ) ) ;
#47974=CIRCLE ( 'NONE', #51224, 9.999999999999998224 ) ;
#48058=DIRECTION ( 'NONE',  ( -0.8660254037844377084, -0.5000000000000015543, -3.252519625699478541E-16 ) ) ;
#48062=VECTOR ( 'NONE', #87336, 1000.000000000000227 ) ;
#48066=CARTESIAN_POINT ( 'NONE',  ( -5.101858724868291617, 167.8615022471904012, 2.586156800657061008E-14 ) ) ;
#48259=CARTESIAN_POINT ( 'NONE',  ( 47.72569090598238972, 198.3615022471903728, 4.570193772333722408E-14 ) ) ;
#48266=CARTESIAN_POINT ( 'NONE',  ( 74.56414817410227158, 187.8759306620403322, 17.47570218321535762 ) ) ;
#48282=( NAMED_UNIT ( * ) PLANE_ANGLE_UNIT ( ) SI_UNIT ( $, .RADIAN. ) );
#48363=UNCERTAINTY_MEASURE_WITH_UNIT (LENGTH_MEASURE( 1.000000000000000082E-05 ), #53726, 'distance_accuracy_value', 'NONE');
#48379=VECTOR ( 'NONE', #26569, 1000.000000000000000 ) ;
#48540=ORIENTED_EDGE ( 'NONE', *, *, #54062, .T. ) ;
#48643=LINE ( 'NONE', #86686, #3795 ) ;
#48831=ADVANCED_FACE ( 'NONE', ( #62033 ), #57635, .F. ) ;
#48903=VERTEX_POINT ( 'NONE', #95008 ) ;
#48931=FACE_OUTER_BOUND ( 'NONE', #92309, .T. ) ;
#48938=FACE_OUTER_BOUND ( 'NONE', #50167, .T. ) ;
#48940=CARTESIAN_POINT ( 'NONE',  ( 46.85966550219794868, 197.8615022471903444, 4.537668576076728569E-14 ) ) ;
#48945=VERTEX_POINT ( 'NONE', #80823 ) ;
#49013=DIRECTION ( 'NONE',  ( -0.8660254037844382635, -0.5000000000000004441, 0.000000000000000000 ) ) ;
#49155=DIRECTION ( 'NONE',  ( 0.8660254037844373753, 0.5000000000000021094, 0.000000000000000000 ) ) ;
#49161=DIRECTION ( 'NONE',  ( -0.8660254037844377084, -0.5000000000000015543, -3.252519625699478541E-16 ) ) ;
#49170=LINE ( 'NONE', #10171, #30235 ) ;
#49218=VECTOR ( 'NONE', #7413, 1000.000000000000114 ) ;
#49606=EDGE_CURVE ( 'NONE', #2096, #89824, #12630, .T. ) ;
#49613=CARTESIAN_POINT ( 'NONE',  ( 52.35966550219797000, 188.3352228055615285, 4.537668576076727938E-14 ) ) ;
#49638=DIRECTION ( 'NONE',  ( 0.8660254037844382635, 0.5000000000000005551, 0.000000000000000000 ) ) ;
#49644=DIRECTION ( 'NONE',  ( 3.755686162884237478E-16, 3.302728788975889054E-33, -1.000000000000000000 ) ) ;
#49651=DIRECTION ( 'NONE',  ( 0.3535533905932792265, -0.6123724356958031301, 0.7071067811865374697 ) ) ;
#49787=ORIENTED_EDGE ( 'NONE', *, *, #21223, .F. ) ;
#49798=AXIS2_PLACEMENT_3D ( 'NONE', #83537, #60668, #91627 ) ;
#49860=EDGE_CURVE ( 'NONE', #78822, #97187, #25193, .T. ) ;
#50080=ORIENTED_EDGE ( 'NONE', *, *, #72324, .T. ) ;
#50167=EDGE_LOOP ( 'NONE', ( #9550, #9475, #29554, #59988 ) ) ;
#50206=CARTESIAN_POINT ( 'NONE',  ( 57.60966550219797000, 179.2419560658249225, 17.47570218321536117 ) ) ;
#50417=ORIENTED_EDGE ( 'NONE', *, *, #53344, .F. ) ;
#50651=EDGE_LOOP ( 'NONE', ( #46396, #51506, #68977 ) ) ;
#50812=DIRECTION ( 'NONE',  ( 1.000000000000000000, 0.000000000000000000, -0.000000000000000000 ) ) ;
#50890=APPLICATION_CONTEXT ( 'automotive_design' ) ;
#50919=EDGE_LOOP ( 'NONE', ( #12540, #92602, #23756 ) ) ;
#51048=AXIS2_PLACEMENT_3D ( 'NONE', #9684, #49651, #32952 ) ;
#51094=AXIS2_PLACEMENT_3D ( 'NONE', #5829, #52419, #4855 ) ;
#51206=DIRECTION ( 'NONE',  ( -0.7886751345948034286, 0.2113248654051702868, 0.5773502691896449379 ) ) ;
#51224=AXIS2_PLACEMENT_3D ( 'NONE', #84409, #32159, #31150 ) ;
#51312=CARTESIAN_POINT ( 'NONE',  ( 42.72569090598236841, 207.0217562850347690, 4.570193772333722408E-14 ) ) ;
#51411=ORIENTED_EDGE ( 'NONE', *, *, #96924, .T. ) ;
#51506=ORIENTED_EDGE ( 'NONE', *, *, #60318, .T. ) ;
#51606=CARTESIAN_POINT ( 'NONE',  ( -10.10185872486829517, 176.5217562850347974, 2.586156800657061008E-14 ) ) ;
#51609=DIRECTION ( 'NONE',  ( 0.000000000000000000, 0.5906904945688776776, -0.8068982213550696114 ) ) ;
#51698=VERTEX_POINT ( 'NONE', #31089 ) ;
#51881=ORIENTED_EDGE ( 'NONE', *, *, #76478, .T. ) ;
#51905=EDGE_CURVE ( 'NONE', #2096, #23710, #49170, .T. ) ;
#51909=DIRECTION ( 'NONE',  ( 0.5000000000000002220, -0.8660254037844384856, -0.000000000000000000 ) ) ;
#51910=ADVANCED_FACE ( 'NONE', ( #95816 ), #57245, .F. ) ;
#52099=CARTESIAN_POINT ( 'NONE',  ( 57.06414817410222895, 218.1868197944957330, 17.47570218321535762 ) ) ;
#52143=EDGE_LOOP ( 'NONE', ( #5684, #31883, #90109, #21878 ) ) ;
#52344=VERTEX_POINT ( 'NONE', #55217 ) ;
#52412=DIRECTION ( 'NONE',  ( -0.5000000000000002220, 0.8660254037844384856, 0.000000000000000000 ) ) ;
#52419=DIRECTION ( 'NONE',  ( -0.7886751345948271874, 0.2113248654051755882, -0.5773502691896106320 ) ) ;
#52462=DIRECTION ( 'NONE',  ( -0.5000000000000019984, 0.8660254037844374864, 0.000000000000000000 ) ) ;
#52699=CIRCLE ( 'NONE', #75379, 3.299999999999998934 ) ;
#52756=EDGE_LOOP ( 'NONE', ( #83614, #78070, #90610, #43421 ) ) ;
#52770=AXIS2_PLACEMENT_3D ( 'NONE', #75004, #5094, #18805 ) ;
#52775=ORIENTED_EDGE ( 'NONE', *, *, #64436, .T. ) ;
#52887=LINE ( 'NONE', #14403, #61274 ) ;
#52935=DIRECTION ( 'NONE',  ( 0.8660254037844394848, 0.4999999999999986122, 0.000000000000000000 ) ) ;
#53050=AXIS2_PLACEMENT_3D ( 'NONE', #75221, #98528, #5804 ) ;
#53152=ORIENTED_EDGE ( 'NONE', *, *, #49606, .F. ) ;
#53344=EDGE_CURVE ( 'NONE', #80748, #53896, #52699, .T. ) ;
#53726=( LENGTH_UNIT ( ) NAMED_UNIT ( * ) SI_UNIT ( .MILLI., .METRE. ) );
#53733=SHAPE_DEFINITION_REPRESENTATION ( #81570, #94304 ) ;
#53749=ORIENTED_EDGE ( 'NONE', *, *, #58963, .T. ) ;
#53896=VERTEX_POINT ( 'NONE', #91135 ) ;
#54062=EDGE_CURVE ( 'NONE', #55615, #19698, #79438, .T. ) ;
#54221=( GEOMETRIC_REPRESENTATION_CONTEXT ( 3 ) GLOBAL_UNCERTAINTY_ASSIGNED_CONTEXT ( ( #1773 ) ) GLOBAL_UNIT_ASSIGNED_CONTEXT ( ( #86839, #48282, #10787 ) ) REPRESENTATION_CONTEXT ( 'NONE', 'WORKASPACE' ) );
#54430=VECTOR ( 'NONE', #17602, 1000.000000000000000 ) ;
#54431=CARTESIAN_POINT ( 'NONE',  ( 63.31414817410234264, 207.3615022471904012, 5.155647304959626021E-14 ) ) ;
#54491=LINE ( 'NONE', #8421, #24756 ) ;
#54578=VECTOR ( 'NONE', #57200, 1000.000000000000114 ) ;
#54693=ADVANCED_FACE ( 'NONE', ( #58767 ), #88257, .F. ) ;
#54700=VECTOR ( 'NONE', #90424, 1000.000000000000114 ) ;
#55204=EDGE_CURVE ( 'NONE', #14940, #12306, #93244, .T. ) ;
#55217=CARTESIAN_POINT ( 'NONE',  ( 41.47569090598247499, 209.1868197944957899, 17.47570218321535762 ) ) ;
#55220=LINE ( 'NONE', #1048, #56284 ) ;
#55404=EDGE_LOOP ( 'NONE', ( #8813, #62447, #34129 ) ) ;
#55615=VERTEX_POINT ( 'NONE', #50206 ) ;
#55692=ORIENTED_EDGE ( 'NONE', *, *, #36398, .F. ) ;
#55694=CARTESIAN_POINT ( 'NONE',  ( 85.72375369157853697, 153.9044130683316212, 0.000000000000000000 ) ) ;
#55797=DIRECTION ( 'NONE',  ( -0.5000000000000002220, 0.8660254037844384856, 0.000000000000000000 ) ) ;
#55992=DIRECTION ( 'NONE',  ( -0.3535533905932733423, 0.6123724356957830350, 0.7071067811865577868 ) ) ;
#56019=ORIENTED_EDGE ( 'NONE', *, *, #7343, .F. ) ;
#56183=AXIS2_PLACEMENT_3D ( 'NONE', #12152, #18757, #49155 ) ;
#56284=VECTOR ( 'NONE', #94777, 1000.000000000000227 ) ;
#56375=ORIENTED_EDGE ( 'NONE', *, *, #37709, .F. ) ;
#56542=STYLED_ITEM('',(#100338),#10898);
#56810=EDGE_CURVE ( 'NONE', #53896, #80748, #9259, .T. ) ;
#56841=CARTESIAN_POINT ( 'NONE',  ( 58.10966550219799132, 178.3759306620403606, -17.47570218321536473 ) ) ;
#57131=VECTOR ( 'NONE', #11778, 1000.000000000000114 ) ;
#57200=DIRECTION ( 'NONE',  ( 0.2588190451025447203, 0.9659258262890618729, 2.299878683274449355E-16 ) ) ;
#57240=CARTESIAN_POINT ( 'NONE',  ( 57.06414817410224316, 218.1868197944957330, -18.47570218321542157 ) ) ;
#57245=PLANE ( 'NONE',  #51048 ) ;
#57283=VECTOR ( 'NONE', #887, 1000.000000000000114 ) ;
#57401=ORIENTED_EDGE ( 'NONE', *, *, #58512, .T. ) ;
#57635=CONICAL_SURFACE ( 'NONE', #77011, 9.999999999999998224, 0.7853981633974214116 ) ;
#57946=ORIENTED_EDGE ( 'NONE', *, *, #17857, .F. ) ;
#58156=DIRECTION ( 'NONE',  ( 0.9659258262890731972, -0.2588190451025028094, 6.018451495431900886E-15 ) ) ;
#58424=EDGE_CURVE ( 'NONE', #48945, #91686, #83780, .T. ) ;
#58440=DIRECTION ( 'NONE',  ( 0.8660254037844375974, 0.5000000000000017764, 3.252519625699413953E-16 ) ) ;
#58493=ORIENTED_EDGE ( 'NONE', *, *, #30280, .T. ) ;
#58512=EDGE_CURVE ( 'NONE', #97187, #48903, #27882, .T. ) ;
#58656=CARTESIAN_POINT ( 'NONE',  ( 58.31414817410232843, 216.0217562850347974, 5.155647304959626021E-14 ) ) ;
#58681=ADVANCED_FACE ( 'NONE', ( #70886 ), #85630, .F. ) ;
#58750=DIRECTION ( 'NONE',  ( 2.816764622163176999E-16, 1.626259812849726945E-16, -1.000000000000000000 ) ) ;
#58760=ORIENTED_EDGE ( 'NONE', *, *, #41746, .F. ) ;
#58767=FACE_OUTER_BOUND ( 'NONE', #28041, .T. ) ;
#58963=EDGE_CURVE ( 'NONE', #81724, #35311, #59648, .T. ) ;
#59036=AXIS2_PLACEMENT_3D ( 'NONE', #29967, #15752, #39042 ) ;
#59163=CARTESIAN_POINT ( 'NONE',  ( 74.93017357788674815, 189.2419560658248940, 5.188172501216619860E-14 ) ) ;
#59174=DIRECTION ( 'NONE',  ( -0.2113248654052096720, -0.7886751345948050940, -0.5773502691896282846 ) ) ;
#59339=CONICAL_SURFACE ( 'NONE', #20559, 9.999999999999998224, 0.7853981633974214116 ) ;
#59587=VERTEX_POINT ( 'NONE', #51312 ) ;
#59615=VECTOR ( 'NONE', #58750, 1000.000000000000000 ) ;
#59648=LINE ( 'NONE', #22666, #47905 ) ;
#59988=ORIENTED_EDGE ( 'NONE', *, *, #1667, .F. ) ;
#60068=FACE_OUTER_BOUND ( 'NONE', #63627, .T. ) ;
#60156=ORIENTED_EDGE ( 'NONE', *, *, #32497, .F. ) ;
#60318=EDGE_CURVE ( 'NONE', #10254, #7154, #62864, .T. ) ;
#60668=DIRECTION ( 'NONE',  ( 0.5000000000000001110, -0.8660254037844384856, -0.000000000000000000 ) ) ;
#60701=CARTESIAN_POINT ( 'NONE',  ( 41.47569090598247499, 209.1868197944957899, 17.47570218321535407 ) ) ;
#60912=CARTESIAN_POINT ( 'NONE',  ( 41.97569090598254604, 208.3207943907112849, 18.47570218321542868 ) ) ;
#61274=VECTOR ( 'NONE', #38165, 1000.000000000000000 ) ;
#61284=VERTEX_POINT ( 'NONE', #41554 ) ;
#61728=CARTESIAN_POINT ( 'NONE',  ( 57.60966550219797000, 179.2419560658249225, 17.47570218321536473 ) ) ;
#61791=DIRECTION ( 'NONE',  ( -2.816764622163176506E-16, -1.626259812849726698E-16, 1.000000000000000000 ) ) ;
#61888=AXIS2_PLACEMENT_3D ( 'NONE', #48259, #78675, #72076 ) ;
#62033=FACE_OUTER_BOUND ( 'NONE', #72989, .T. ) ;
#62125=ADVANCED_FACE ( 'NONE', ( #48938 ), #10436, .F. ) ;
#62282=PLANE ( 'NONE',  #97812 ) ;
#62298=EDGE_CURVE ( 'NONE', #45554, #51698, #4141, .T. ) ;
#62447=ORIENTED_EDGE ( 'NONE', *, *, #25630, .T. ) ;
#62712=AXIS2_PLACEMENT_3D ( 'NONE', #66787, #30281, #77392 ) ;
#62800=VECTOR ( 'NONE', #52412, 1000.000000000000227 ) ;
#62857=ORIENTED_EDGE ( 'NONE', *, *, #21528, .T. ) ;
#62864=LINE ( 'NONE', #71495, #65839 ) ;
#62909=CARTESIAN_POINT ( 'NONE',  ( 65.36586985908992631, 182.5653022007868458, 0.000000000000000000 ) ) ;
#63114=DIRECTION ( 'NONE',  ( 3.755686162884236985E-16, -2.795463207713249976E-32, -1.000000000000000000 ) ) ;
#63165=LINE ( 'NONE', #47951, #25149 ) ;
#63430=CARTESIAN_POINT ( 'NONE',  ( 58.97569090598252473, 178.8759306620404175, 18.47570218321542868 ) ) ;
#63455=CARTESIAN_POINT ( 'NONE',  ( 40.60966550219796289, 208.6868197944957330, 17.47570218321536473 ) ) ;
#63466=DIRECTION ( 'NONE',  ( -0.2588190451025239591, -0.9659258262890673130, -6.735114559760606617E-15 ) ) ;
#63627=EDGE_LOOP ( 'NONE', ( #44162, #34018, #19949 ) ) ;
#63997=LINE ( 'NONE', #86361, #28159 ) ;
#64055=ORIENTED_EDGE ( 'NONE', *, *, #36522, .T. ) ;
#64168=ADVANCED_FACE ( 'NONE', ( #34704, #42786 ), #73720, .T. ) ;
#64171=DIRECTION ( 'NONE',  ( -0.3535533905932763954, 0.6123724356958081261, 0.7071067811865344721 ) ) ;
#64317=LINE ( 'NONE', #11140, #54578 ) ;
#64402=VECTOR ( 'NONE', #63466, 1000.000000000000114 ) ;
#64436=EDGE_CURVE ( 'NONE', #89824, #20684, #9375, .T. ) ;
#64559=EDGE_CURVE ( 'NONE', #78822, #81724, #29623, .T. ) ;
#64614=LINE ( 'NONE', #95569, #26675 ) ;
#64696=DIRECTION ( 'NONE',  ( -0.5000000000000002220, 0.8660254037844384856, 0.000000000000000000 ) ) ;
#64753=ADVANCED_FACE ( 'NONE', ( #45672 ), #66504, .T. ) ;
#64846=VECTOR ( 'NONE', #98401, 1000.000000000000000 ) ;
#65203=LINE ( 'NONE', #85172, #69386 ) ;
#65412=APPLICATION_CONTEXT ( 'automotive_design' ) ;
#65535=EDGE_CURVE ( 'NONE', #7154, #55615, #9464, .T. ) ;
#65653=PLANE ( 'NONE',  #94741 ) ;
#65839=VECTOR ( 'NONE', #94810, 1000.000000000000114 ) ;
#65931=ADVANCED_FACE ( 'NONE', ( #11557 ), #12047, .T. ) ;
#66002=AXIS2_PLACEMENT_3D ( 'NONE', #48940, #73737, #66127 ) ;
#66077=LINE ( 'NONE', #36653, #54700 ) ;
#66127=DIRECTION ( 'NONE',  ( -0.5000000000000002220, 0.8660254037844384856, 0.000000000000000000 ) ) ;
#66137=PLANE ( 'NONE',  #51094 ) ;
#66205=ADVANCED_FACE ( 'NONE', ( #86477 ), #1327, .T. ) ;
#66238=DIRECTION ( 'NONE',  ( -0.5906904945688911113, 0.000000000000000000, -0.8068982213550597304 ) ) ;
#66271=EDGE_LOOP ( 'NONE', ( #47100, #22057, #49787, #32347 ) ) ;
#66504=PLANE ( 'NONE',  #27253 ) ;
#66648=EDGE_CURVE ( 'NONE', #76155, #22001, #11326, .T. ) ;
#66787=CARTESIAN_POINT ( 'NONE',  ( 63.31414817410235685, 207.3615022471904012, 5.155647304959626652E-14 ) ) ;
#67001=EDGE_CURVE ( 'NONE', #82304, #10254, #19791, .T. ) ;
#67040=DIRECTION ( 'NONE',  ( -0.3535533905932853327, 0.6123724356958029080, -0.7071067811865343611 ) ) ;
#67185=AXIS2_PLACEMENT_3D ( 'NONE', #90076, #27746, #12552 ) ;
#67294=FACE_OUTER_BOUND ( 'NONE', #15540, .T. ) ;
#67416=CARTESIAN_POINT ( 'NONE',  ( 57.60966550219797710, 179.2419560658249225, -17.47570218321534696 ) ) ;
#67583=LINE ( 'NONE', #75703, #445 ) ;
#67689=DIRECTION ( 'NONE',  ( 0.7886751345947972114, -0.2113248654051897435, 0.5773502691896462702 ) ) ;
#67808=CARTESIAN_POINT ( 'NONE',  ( 58.47569090598246788, 179.7419560658249509, -18.47570218321542868 ) ) ;
#68131=EDGE_LOOP ( 'NONE', ( #5572, #70773, #93546 ) ) ;
#68784=AXIS2_PLACEMENT_3D ( 'NONE', #15354, #91924, #23457 ) ;
#68976=CYLINDRICAL_SURFACE ( 'NONE', #80183, 3.300000000000010925 ) ;
#68977=ORIENTED_EDGE ( 'NONE', *, *, #81676, .F. ) ;
#69386=VECTOR ( 'NONE', #49013, 1000.000000000000227 ) ;
#69531=ORIENTED_EDGE ( 'NONE', *, *, #85458, .T. ) ;
#69548=MECHANICAL_DESIGN_GEOMETRIC_PRESENTATION_REPRESENTATION('',(#56542),#4);
#69754=ORIENTED_EDGE ( 'NONE', *, *, #13245, .F. ) ;
#70041=DIRECTION ( 'NONE',  ( 0.8660254037844382635, 0.5000000000000004441, 0.000000000000000000 ) ) ;
#70084=PLANE ( 'NONE',  #81502 ) ;
#70099=VERTEX_POINT ( 'NONE', #33040 ) ;
#70118=CARTESIAN_POINT ( 'NONE',  ( 68.31414817410238527, 198.7012482093460335, 5.278111984874363062E-14 ) ) ;
#70361=DIRECTION ( 'NONE',  ( 0.5000000000000009992, -0.8660254037844380415, 0.000000000000000000 ) ) ;
#70516=LINE ( 'NONE', #76628, #96418 ) ;
#70529=EDGE_CURVE ( 'NONE', #70099, #35311, #11174, .T. ) ;
#70773=ORIENTED_EDGE ( 'NONE', *, *, #20301, .T. ) ;
#70882=ORIENTED_EDGE ( 'NONE', *, *, #2733, .T. ) ;
#70886=FACE_OUTER_BOUND ( 'NONE', #31485, .T. ) ;
#71010=ADVANCED_FACE ( 'NONE', ( #95697 ), #26244, .F. ) ;
#71081=EDGE_CURVE ( 'NONE', #81724, #45554, #52887, .T. ) ;
#71260=EDGE_CURVE ( 'NONE', #76155, #35311, #77530, .T. ) ;
#71393=DIRECTION ( 'NONE',  ( -0.4999999999999997224, 0.8660254037844387076, 0.000000000000000000 ) ) ;
#71495=CARTESIAN_POINT ( 'NONE',  ( 58.29267820409022960, 179.0589433639326558, -17.47570218321535762 ) ) ;
#71626=CIRCLE ( 'NONE', #61888, 9.999999999999998224 ) ;
#71745=CARTESIAN_POINT ( 'NONE',  ( 41.47569090598248920, 209.1868197944957899, -17.47570218321533275 ) ) ;
#71773=LINE ( 'NONE', #24644, #98337 ) ;
#71776=CARTESIAN_POINT ( 'NONE',  ( 57.60966550219796289, 179.2419560658249225, 18.47570218321542868 ) ) ;
#71920=DIRECTION ( 'NONE',  ( -0.2588190451025411121, -0.9659258262890628721, -2.299878683274462667E-16 ) ) ;
#72076=DIRECTION ( 'NONE',  ( -0.5000000000000019984, 0.8660254037844374864, 0.000000000000000000 ) ) ;
#72272=EDGE_LOOP ( 'NONE', ( #29481, #14708, #84966 ) ) ;
#72283=DIRECTION ( 'NONE',  ( 0.8660254037844394848, 0.4999999999999986122, 0.000000000000000000 ) ) ;
#72324=EDGE_CURVE ( 'NONE', #10254, #1997, #42630, .T. ) ;
#72421=AXIS2_PLACEMENT_3D ( 'NONE', #62909, #46709, #31007 ) ;
#72432=AXIS2_PLACEMENT_3D ( 'NONE', #25311, #40989, #72945 ) ;
#72445=PLANE ( 'NONE',  #72432 ) ;
#72493=CARTESIAN_POINT ( 'NONE',  ( 58.47569090598246078, 179.7419560658249509, -18.47570218321543223 ) ) ;
#72504=ORIENTED_EDGE ( 'NONE', *, *, #51905, .T. ) ;
#72626=DIRECTION ( 'NONE',  ( -0.8660254037844382635, -0.5000000000000004441, -1.232595164407830946E-32 ) ) ;
#72685=VECTOR ( 'NONE', #20095, 1000.000000000000000 ) ;
#72732=CARTESIAN_POINT ( 'NONE',  ( 58.00798602660123038, 188.7095308348468734, 4.041334437186271426E-16 ) ) ;
#72945=DIRECTION ( 'NONE',  ( -0.5000000000000002220, 0.8660254037844384856, 0.000000000000000000 ) ) ;
#72989=EDGE_LOOP ( 'NONE', ( #44944, #696, #16071, #80935 ) ) ;
#73114=ORIENTED_EDGE ( 'NONE', *, *, #5791, .T. ) ;
#73119=ORIENTED_EDGE ( 'NONE', *, *, #37503, .T. ) ;
#73145=EDGE_CURVE ( 'NONE', #70099, #15824, #76678, .T. ) ;
#73198=ORIENTED_EDGE ( 'NONE', *, *, #92136, .T. ) ;
#73309=ADVANCED_FACE ( 'NONE', ( #48931 ), #10431, .T. ) ;
#73349=DIRECTION ( 'NONE',  ( 0.7886751345947996539, -0.2113248654051860242, -0.5773502691896443828 ) ) ;
#73694=CARTESIAN_POINT ( 'NONE',  ( 58.97569090598252473, 178.8759306620404175, -17.47570218321536473 ) ) ;
#73720=PLANE ( 'NONE',  #53050 ) ;
#73737=DIRECTION ( 'NONE',  ( 0.8660254037844384856, 0.5000000000000002220, 3.252519625699449945E-16 ) ) ;
#73753=ORIENTED_EDGE ( 'NONE', *, *, #58963, .F. ) ;
#74090=ORIENTED_EDGE ( 'NONE', *, *, #5255, .T. ) ;
#74436=DIRECTION ( 'NONE',  ( 0.8660254037844384856, 0.5000000000000002220, 3.252519625699449945E-16 ) ) ;
#74475=VERTEX_POINT ( 'NONE', #47684 ) ;
#75000=DIRECTION ( 'NONE',  ( -0.8660254037844382635, -0.5000000000000005551, 0.000000000000000000 ) ) ;
#75004=CARTESIAN_POINT ( 'NONE',  ( 138.1418008908465822, 79.75620593067000641, -17.47570218321536473 ) ) ;
#75114=DIRECTION ( 'NONE',  ( 0.5000000000000001110, -0.8660254037844384856, -0.000000000000000000 ) ) ;
#75221=CARTESIAN_POINT ( 'NONE',  ( 58.10966550219799132, 178.3759306620403606, -18.47570218321542868 ) ) ;
#75361=VECTOR ( 'NONE', #10583, 1000.000000000000114 ) ;
#75379=AXIS2_PLACEMENT_3D ( 'NONE', #19488, #27063, #4763 ) ;
#75437=AXIS2_PLACEMENT_3D ( 'NONE', #20949, #82279, #72283 ) ;
#75703=CARTESIAN_POINT ( 'NONE',  ( 74.56414817410228579, 187.8759306620403322, -18.47570218321542157 ) ) ;
#75983=CARTESIAN_POINT ( 'NONE',  ( 40.60966550219796289, 208.6868197944957330, 17.47570218321535762 ) ) ;
#76106=LINE ( 'NONE', #91811, #64846 ) ;
#76155=VERTEX_POINT ( 'NONE', #82559 ) ;
#76174=ADVANCED_FACE ( 'NONE', ( #67294 ), #97723, .F. ) ;
#76242=ORIENTED_EDGE ( 'NONE', *, *, #62298, .T. ) ;
#76300=CARTESIAN_POINT ( 'NONE',  ( 63.72375369157849434, 192.0095308348468564, 0.000000000000000000 ) ) ;
#76412=PLANE ( 'NONE',  #34654 ) ;
#76478=EDGE_CURVE ( 'NONE', #77213, #76155, #26365, .T. ) ;
#76628=CARTESIAN_POINT ( 'NONE',  ( 41.47569090598247499, 209.1868197944957899, 18.47570218321542868 ) ) ;
#76678=LINE ( 'NONE', #84810, #100213 ) ;
#77011=AXIS2_PLACEMENT_3D ( 'NONE', #54431, #46858, #52462 ) ;
#77143=ADVANCED_FACE ( 'NONE', ( #81549 ), #90147, .T. ) ;
#77213=VERTEX_POINT ( 'NONE', #52099 ) ;
#77392=DIRECTION ( 'NONE',  ( -0.5000000000000019984, 0.8660254037844374864, 0.000000000000000000 ) ) ;
#77530=LINE ( 'NONE', #86175, #43487 ) ;
#77533=EDGE_CURVE ( 'NONE', #59587, #20684, #66077, .T. ) ;
#77536=CARTESIAN_POINT ( 'NONE',  ( 41.47569090598247499, 209.1868197944957899, 17.47570218321535762 ) ) ;
#77650=FACE_OUTER_BOUND ( 'NONE', #46554, .T. ) ;
#77920=CARTESIAN_POINT ( 'NONE',  ( 52.35966550219796289, 188.3352228055615001, 4.537668576076727307E-14 ) ) ;
#78070=ORIENTED_EDGE ( 'NONE', *, *, #1667, .T. ) ;
#78485=FACE_OUTER_BOUND ( 'NONE', #18809, .T. ) ;
#78566=AXIS2_PLACEMENT_3D ( 'NONE', #80460, #25729, #94651 ) ;
#78632=CIRCLE ( 'NONE', #34917, 3.299999999999978950 ) ;
#78675=DIRECTION ( 'NONE',  ( -0.8660254037844379305, -0.5000000000000016653, -3.252519625699479034E-16 ) ) ;
#78771=PRODUCT_DEFINITION_CONTEXT ( 'detailed design', #50890, 'design' ) ;
#78822=VERTEX_POINT ( 'NONE', #23377 ) ;
#78903=CARTESIAN_POINT ( 'NONE',  ( 58.68017357788676946, 217.3877816888190750, 5.188172501216618598E-14 ) ) ;
#79383=ORIENTED_EDGE ( 'NONE', *, *, #7343, .T. ) ;
#79438=LINE ( 'NONE', #8987, #2702 ) ;
#79698=CARTESIAN_POINT ( 'NONE',  ( 138.1418008908465822, 79.75620593067000641, 17.47570218321536117 ) ) ;
#80183=AXIS2_PLACEMENT_3D ( 'NONE', #29008, #75114, #29983 ) ;
#80243=ORIENTED_EDGE ( 'NONE', *, *, #65535, .F. ) ;
#80279=ORIENTED_EDGE ( 'NONE', *, *, #71260, .F. ) ;
#80448=CARTESIAN_POINT ( 'NONE',  ( 41.10966550219802684, 207.8207943907112565, 17.47570218321536117 ) ) ;
#80460=CARTESIAN_POINT ( 'NONE',  ( 47.72569090598238972, 198.3615022471903728, 4.570193772333722408E-14 ) ) ;
#80748=VERTEX_POINT ( 'NONE', #17273 ) ;
#80811=CIRCLE ( 'NONE', #93501, 10.99999999999989164 ) ;
#80823=CARTESIAN_POINT ( 'NONE',  ( 69.68017357788663446, 198.3352228055616706, 5.322883649122824736E-14 ) ) ;
#80935=ORIENTED_EDGE ( 'NONE', *, *, #58424, .F. ) ;
#81008=CARTESIAN_POINT ( 'NONE',  ( 74.06414817410222895, 188.7419560658248656, -18.47570218321542868 ) ) ;
#81153=CARTESIAN_POINT ( 'NONE',  ( 57.74716087599451697, 218.0038070926034948, -17.47570218321534341 ) ) ;
#81502=AXIS2_PLACEMENT_3D ( 'NONE', #7804, #31085, #93942 ) ;
#81549=FACE_OUTER_BOUND ( 'NONE', #50651, .T. ) ;
#81570=PRODUCT_DEFINITION_SHAPE ( 'NONE', 'NONE',  #21642 ) ;
#81583=CYLINDRICAL_SURFACE ( 'NONE', #56183, 3.300000000000010925 ) ;
#81611=CARTESIAN_POINT ( 'NONE',  ( 58.97569090598252473, 178.8759306620404175, -18.47570218321542868 ) ) ;
#81676=EDGE_CURVE ( 'NONE', #48903, #7154, #24366, .T. ) ;
#81724=VERTEX_POINT ( 'NONE', #33985 ) ;
#81895=AXIS2_PLACEMENT_3D ( 'NONE', #20173, #35853, #4970 ) ;
#81933=CARTESIAN_POINT ( 'NONE',  ( 74.56414817410227158, 187.8759306620403322, 17.47570218321536473 ) ) ;
#82024=CONICAL_SURFACE ( 'NONE', #41543, 11.00000000000002842, 0.7853981633974557175 ) ;
#82279=DIRECTION ( 'NONE',  ( 0.5000000000000002220, -0.8660254037844387076, -0.000000000000000000 ) ) ;
#82304=VERTEX_POINT ( 'NONE', #42253 ) ;
#82559=CARTESIAN_POINT ( 'NONE',  ( 57.06414817410224316, 218.1868197944957330, -17.47570218321533631 ) ) ;
#82613=ORIENTED_EDGE ( 'NONE', *, *, #71260, .T. ) ;
#82768=CARTESIAN_POINT ( 'NONE',  ( 58.10966550219799132, 178.3759306620403606, 18.47570218321542868 ) ) ;
#83476=VECTOR ( 'NONE', #28390, 999.9999999999998863 ) ;
#83512=PRODUCT_DEFINITION_FORMATION_WITH_SPECIFIED_SOURCE ( 'ANY', '', #13637, .NOT_KNOWN. ) ;
#83537=CARTESIAN_POINT ( 'NONE',  ( 60.86586985908987657, 190.3595308348468791, 0.000000000000000000 ) ) ;
#83569=VECTOR ( 'NONE', #11143, 1000.000000000000114 ) ;
#83614=ORIENTED_EDGE ( 'NONE', *, *, #9846, .T. ) ;
#83685=DIRECTION ( 'NONE',  ( 0.8660254037844385966, 0.5000000000000003331, 3.252519625699449945E-16 ) ) ;
#83712=DIRECTION ( 'NONE',  ( 0.8660254037844382635, 0.5000000000000005551, 0.000000000000000000 ) ) ;
#83780=CIRCLE ( 'NONE', #43305, 10.99999999999989164 ) ;
#83938=DIRECTION ( 'NONE',  ( 0.5000000000000002220, -0.8660254037844385966, 0.000000000000000000 ) ) ;
#83971=CARTESIAN_POINT ( 'NONE',  ( 58.47569090598247499, 179.7419560658249509, -18.47570218321543223 ) ) ;
#84048=DIRECTION ( 'NONE',  ( 0.8660254037844382635, 0.5000000000000004441, 0.000000000000000000 ) ) ;
#84098=ORIENTED_EDGE ( 'NONE', *, *, #44935, .T. ) ;
#84217=LINE ( 'NONE', #14270, #29592 ) ;
#84357=CARTESIAN_POINT ( 'NONE',  ( 138.1418008908465822, 79.75620593067000641, -17.47570218321535052 ) ) ;
#84409=CARTESIAN_POINT ( 'NONE',  ( 63.31414817410235685, 207.3615022471904012, 5.155647304959626652E-14 ) ) ;
#84534=FACE_OUTER_BOUND ( 'NONE', #55404, .T. ) ;
#84677=CARTESIAN_POINT ( 'NONE',  ( 120.8212928151578041, 69.75620593067000641, 5.188172501216618598E-14 ) ) ;
#84810=CARTESIAN_POINT ( 'NONE',  ( 41.54267820409027934, 208.0707943907112849, -17.97570218321537894 ) ) ;
#84966=ORIENTED_EDGE ( 'NONE', *, *, #6347, .F. ) ;
#85172=CARTESIAN_POINT ( 'NONE',  ( 58.10966550219799132, 178.3759306620403606, 17.47570218321536473 ) ) ;
#85458=EDGE_CURVE ( 'NONE', #51698, #78822, #76106, .T. ) ;
#85630=CYLINDRICAL_SURFACE ( 'NONE', #28783, 10.00000000000001421 ) ;
#86152=CARTESIAN_POINT ( 'NONE',  ( 57.56414817410228579, 217.3207943907112281, -18.47570218321542868 ) ) ;
#86175=CARTESIAN_POINT ( 'NONE',  ( 57.56414817410227158, 217.3207943907112281, -18.47570218321543578 ) ) ;
#86361=CARTESIAN_POINT ( 'NONE',  ( 41.47569090598248920, 209.1868197944957899, -18.47570218321542868 ) ) ;
#86477=FACE_OUTER_BOUND ( 'NONE', #33668, .T. ) ;
#86567=AXIS2_PLACEMENT_3D ( 'NONE', #34451, #49161, #88713 ) ;
#86637=ORIENTED_EDGE ( 'NONE', *, *, #20531, .F. ) ;
#86683=DIRECTION ( 'NONE',  ( 0.5000000000000001110, -0.8660254037844384856, -0.000000000000000000 ) ) ;
#86686=CARTESIAN_POINT ( 'NONE',  ( 58.10966550219803395, 178.3759306620403891, -17.47570218321534696 ) ) ;
#86839=( LENGTH_UNIT ( ) NAMED_UNIT ( * ) SI_UNIT ( .MILLI., .METRE. ) );
#86963=ORIENTED_EDGE ( 'NONE', *, *, #67001, .F. ) ;
#86997=CARTESIAN_POINT ( 'NONE',  ( 57.60966550219794158, 179.2419560658248940, 18.47570218321542868 ) ) ;
#87070=CARTESIAN_POINT ( 'NONE',  ( 74.49716087599449565, 188.9919560658248656, -17.97570218321539315 ) ) ;
#87336=DIRECTION ( 'NONE',  ( 0.5000000000000002220, -0.8660254037844384856, 0.000000000000000000 ) ) ;
#87339=FACE_OUTER_BOUND ( 'NONE', #52143, .T. ) ;
#87898=ORIENTED_EDGE ( 'NONE', *, *, #17857, .T. ) ;
#88018=ORIENTED_EDGE ( 'NONE', *, *, #92136, .F. ) ;
#88257=PLANE ( 'NONE',  #52770 ) ;
#88305=CIRCLE ( 'NONE', #78566, 9.999999999999998224 ) ;
#88479=ORIENTED_EDGE ( 'NONE', *, *, #51905, .F. ) ;
#88713=DIRECTION ( 'NONE',  ( 0.5000000000000009992, -0.8660254037844380415, 0.000000000000000000 ) ) ;
#88828=ADVANCED_BREP_SHAPE_REPRESENTATION ( '', ( #10898, #68784 ), #54221 ) ;
#89010=EDGE_LOOP ( 'NONE', ( #9941, #29344, #82613, #23534 ) ) ;
#89091=ORIENTED_EDGE ( 'NONE', *, *, #3217, .T. ) ;
#89290=DIRECTION ( 'NONE',  ( 0.5906904945688895570, 0.000000000000000000, 0.8068982213550607296 ) ) ;
#89824=VERTEX_POINT ( 'NONE', #77920 ) ;
#90041=CARTESIAN_POINT ( 'NONE',  ( 58.97569090598253183, 178.8759306620404175, 18.47570218321542868 ) ) ;
#90076=CARTESIAN_POINT ( 'NONE',  ( 46.85966550219794868, 197.8615022471903444, 4.537668576076728569E-14 ) ) ;
#90109=ORIENTED_EDGE ( 'NONE', *, *, #36522, .F. ) ;
#90137=DIRECTION ( 'NONE',  ( -0.9659258262890674240, 0.2588190451025240146, -2.299878683274403996E-16 ) ) ;
#90147=PLANE ( 'NONE',  #27191 ) ;
#90424=DIRECTION ( 'NONE',  ( -0.9659258262890667579, 0.2588190451025264016, -1.433922627038915147E-16 ) ) ;
#90610=ORIENTED_EDGE ( 'NONE', *, *, #41746, .T. ) ;
#90798=FACE_OUTER_BOUND ( 'NONE', #92355, .T. ) ;
#90819=ORIENTED_EDGE ( 'NONE', *, *, #67001, .T. ) ;
#91039=VECTOR ( 'NONE', #22541, 999.9999999999998863 ) ;
#91068=ORIENTED_EDGE ( 'NONE', *, *, #66648, .T. ) ;
#91135=CARTESIAN_POINT ( 'NONE',  ( 62.50798602660128012, 180.9153022007868401, 4.041334437186263538E-16 ) ) ;
#91279=DIRECTION ( 'NONE',  ( 0.9659258262890757507, -0.2588190451024926508, 3.165834739509918729E-16 ) ) ;
#91627=DIRECTION ( 'NONE',  ( 0.8660254037844394848, 0.4999999999999986122, 0.000000000000000000 ) ) ;
#91630=CARTESIAN_POINT ( 'NONE',  ( 58.10966550219799132, 178.3759306620403606, -17.47570218321536473 ) ) ;
#91686=VERTEX_POINT ( 'NONE', #78903 ) ;
#91778=LINE ( 'NONE', #22837, #34511 ) ;
#91811=CARTESIAN_POINT ( 'NONE',  ( 74.93017357788674815, 189.2419560658248940, 5.188172501216619860E-14 ) ) ;
#91855=AXIS2_PLACEMENT_3D ( 'NONE', #86997, #17525, #28616 ) ;
#91924=DIRECTION ( 'NONE',  ( 0.000000000000000000, 0.000000000000000000, 1.000000000000000000 ) ) ;
#91994=CARTESIAN_POINT ( 'NONE',  ( 41.10966550219804816, 207.8207943907112565, -18.47570218321542868 ) ) ;
#92124=VERTEX_POINT ( 'NONE', #36734 ) ;
#92136=EDGE_CURVE ( 'NONE', #35311, #97187, #14923, .T. ) ;
#92271=DIRECTION ( 'NONE',  ( -0.8660254037844382635, -0.5000000000000005551, 0.000000000000000000 ) ) ;
#92309=EDGE_LOOP ( 'NONE', ( #32222, #95592, #29624, #13559 ) ) ;
#92335=DIRECTION ( 'NONE',  ( -0.8660254037844384856, -0.5000000000000002220, -3.252519625699449945E-16 ) ) ;
#92355=EDGE_LOOP ( 'NONE', ( #48540, #20821, #4726, #17925 ) ) ;
#92389=EDGE_LOOP ( 'NONE', ( #64055, #24625, #3493 ) ) ;
#92602=ORIENTED_EDGE ( 'NONE', *, *, #13227, .T. ) ;
#93244=CIRCLE ( 'NONE', #75437, 3.299999999999978950 ) ;
#93501=AXIS2_PLACEMENT_3D ( 'NONE', #43477, #26799, #27303 ) ;
#93546=ORIENTED_EDGE ( 'NONE', *, *, #19671, .T. ) ;
#93867=DIRECTION ( 'NONE',  ( -3.755686162884237478E-16, -3.302728788975889054E-33, 1.000000000000000000 ) ) ;
#93942=DIRECTION ( 'NONE',  ( -3.755686162884236985E-16, 2.795463207713249976E-32, 1.000000000000000000 ) ) ;
#94264=LINE ( 'NONE', #55694, #35419 ) ;
#94304=SHAPE_REPRESENTATION ( 'Screw Retaining Piece Part', ( #68784 ), #54221 ) ;
#94336=PLANE ( 'NONE',  #12113 ) ;
#94368=DIRECTION ( 'NONE',  ( -0.6123724356957923609, -0.3535533905932727317, 0.7071067811865499042 ) ) ;
#94508=EDGE_CURVE ( 'NONE', #12322, #51698, #54491, .T. ) ;
#94651=DIRECTION ( 'NONE',  ( -0.5000000000000019984, 0.8660254037844374864, 0.000000000000000000 ) ) ;
#94741=AXIS2_PLACEMENT_3D ( 'NONE', #20076, #4360, #42834 ) ;
#94751=AXIS2_PLACEMENT_3D ( 'NONE', #82768, #29029, #50812 ) ;
#94777=DIRECTION ( 'NONE',  ( 0.5000000000000001110, -0.8660254037844384856, -0.000000000000000000 ) ) ;
#94780=ADVANCED_FACE ( 'NONE', ( #1205 ), #70084, .F. ) ;
#94810=DIRECTION ( 'NONE',  ( -0.9659258262890627611, 0.2588190451025410566, 1.149007080238459400E-14 ) ) ;
#94819=ORIENTED_EDGE ( 'NONE', *, *, #53344, .T. ) ;
#94938=DIRECTION ( 'NONE',  ( -0.5000000000000002220, 0.8660254037844385966, 0.000000000000000000 ) ) ;
#95008=CARTESIAN_POINT ( 'NONE',  ( 58.47569090598246788, 179.7419560658249509, -18.47570218321542868 ) ) ;
#95060=AXIS2_PLACEMENT_3D ( 'NONE', #81933, #67689, #36781 ) ;
#95345=AXIS2_PLACEMENT_3D ( 'NONE', #5310, #13419, #51909 ) ;
#95569=CARTESIAN_POINT ( 'NONE',  ( 74.56414817410225737, 187.8759306620403322, 18.47570218321542868 ) ) ;
#95592=ORIENTED_EDGE ( 'NONE', *, *, #13893, .F. ) ;
#95613=ADVANCED_FACE ( 'NONE', ( #87339 ), #8263, .F. ) ;
#95697=FACE_OUTER_BOUND ( 'NONE', #31892, .T. ) ;
#95802=FACE_OUTER_BOUND ( 'NONE', #99345, .T. ) ;
#95816=FACE_OUTER_BOUND ( 'NONE', #89010, .T. ) ;
#95852=ORIENTED_EDGE ( 'NONE', *, *, #12683, .F. ) ;
#96006=ORIENTED_EDGE ( 'NONE', *, *, #64559, .F. ) ;
#96360=ORIENTED_EDGE ( 'NONE', *, *, #62298, .F. ) ;
#96400=LINE ( 'NONE', #34558, #57131 ) ;
#96408=EDGE_CURVE ( 'NONE', #48903, #10254, #46402, .T. ) ;
#96418=VECTOR ( 'NONE', #93867, 1000.000000000000000 ) ;
#96641=DIRECTION ( 'NONE',  ( 0.8660254037844394848, 0.4999999999999986122, 0.000000000000000000 ) ) ;
#96704=LINE ( 'NONE', #27273, #36633 ) ;
#96732=VECTOR ( 'NONE', #75000, 1000.000000000000114 ) ;
#96780=VECTOR ( 'NONE', #29819, 1000.000000000000114 ) ;
#96814=VECTOR ( 'NONE', #55992, 1000.000000000000000 ) ;
#96924=EDGE_CURVE ( 'NONE', #48903, #70099, #63997, .T. ) ;
#96927=AXIS2_PLACEMENT_3D ( 'NONE', #9419, #32208, #63114 ) ;
#97187=VERTEX_POINT ( 'NONE', #81008 ) ;
#97295=ORIENTED_EDGE ( 'NONE', *, *, #85458, .F. ) ;
#97723=PLANE ( 'NONE',  #27121 ) ;
#97769=LINE ( 'NONE', #61728, #6869 ) ;
#97812=AXIS2_PLACEMENT_3D ( 'NONE', #23795, #71920, #61791 ) ;
#97841=FACE_OUTER_BOUND ( 'NONE', #98166, .T. ) ;
#98166=EDGE_LOOP ( 'NONE', ( #84098, #89091, #56019 ) ) ;
#98337=VECTOR ( 'NONE', #1362, 1000.000000000000227 ) ;
#98367=FACE_BOUND ( 'NONE', #27676, .T. ) ;
#98401=DIRECTION ( 'NONE',  ( 2.816764622163176506E-16, 1.626259812849726205E-16, -1.000000000000000000 ) ) ;
#98515=ORIENTED_EDGE ( 'NONE', *, *, #94508, .T. ) ;
#98528=DIRECTION ( 'NONE',  ( 0.5000000000000005551, -0.8660254037844383745, 0.000000000000000000 ) ) ;
#98551=ORIENTED_EDGE ( 'NONE', *, *, #64559, .T. ) ;
#98626=AXIS2_PLACEMENT_3D ( 'NONE', #2851, #11451, #42306 ) ;
#98645=VECTOR ( 'NONE', #10671, 1000.000000000000114 ) ;
#98678=PLANE ( 'NONE',  #81895 ) ;
#98816=ORIENTED_EDGE ( 'NONE', *, *, #64436, .F. ) ;
#98893=CYLINDRICAL_SURFACE ( 'NONE', #59036, 10.00000000000001421 ) ;
#98915=DIRECTION ( 'NONE',  ( -0.4999999999999996669, 0.8660254037844387076, 0.000000000000000000 ) ) ;
#99104=PLANE ( 'NONE',  #95060 ) ;
#99146=ADVANCED_FACE ( 'NONE', ( #25872 ), #25037, .F. ) ;
#99233=CARTESIAN_POINT ( 'NONE',  ( 63.72375369157850855, 192.0095308348468564, 0.000000000000000000 ) ) ;
#99259=DIRECTION ( 'NONE',  ( 0.6123724356957995774, 0.3535533905932699006, 0.7071067811865450192 ) ) ;
#99345=EDGE_LOOP ( 'NONE', ( #34350, #23119, #2083, #95852 ) ) ;
#99445=ADVANCED_FACE ( 'NONE', ( #33505 ), #94336, .T. ) ;
#99493=DIRECTION ( 'NONE',  ( -0.6123724356957759296, -0.3535533905932816134, 0.7071067811865596742 ) ) ;
#99612=LINE ( 'NONE', #90041, #99964 ) ;
#99763=ORIENTED_EDGE ( 'NONE', *, *, #99917, .T. ) ;
#99792=AXIS2_PLACEMENT_3D ( 'NONE', #45331, #37238, #52935 ) ;
#99917=EDGE_CURVE ( 'NONE', #2096, #59587, #88305, .T. ) ;
#99964=VECTOR ( 'NONE', #83938, 999.9999999999998863 ) ;
#100213=VECTOR ( 'NONE', #99493, 1000.000000000000000 ) ;
#100332=COLOUR_RGB('Black',0.12,0.14,0.17);
#100333=FILL_AREA_STYLE_COLOUR('',#100332);
#100334=FILL_AREA_STYLE('',(#100333));
#100335=SURFACE_STYLE_FILL_AREA(#100334);
#100336=SURFACE_SIDE_STYLE('',(#100335));
#100337=SURFACE_STYLE_USAGE(.BOTH.,#100336);
#100338=PRESENTATION_STYLE_ASSIGNMENT((#100337));
ENDSEC;
END-ISO-10303-21;
